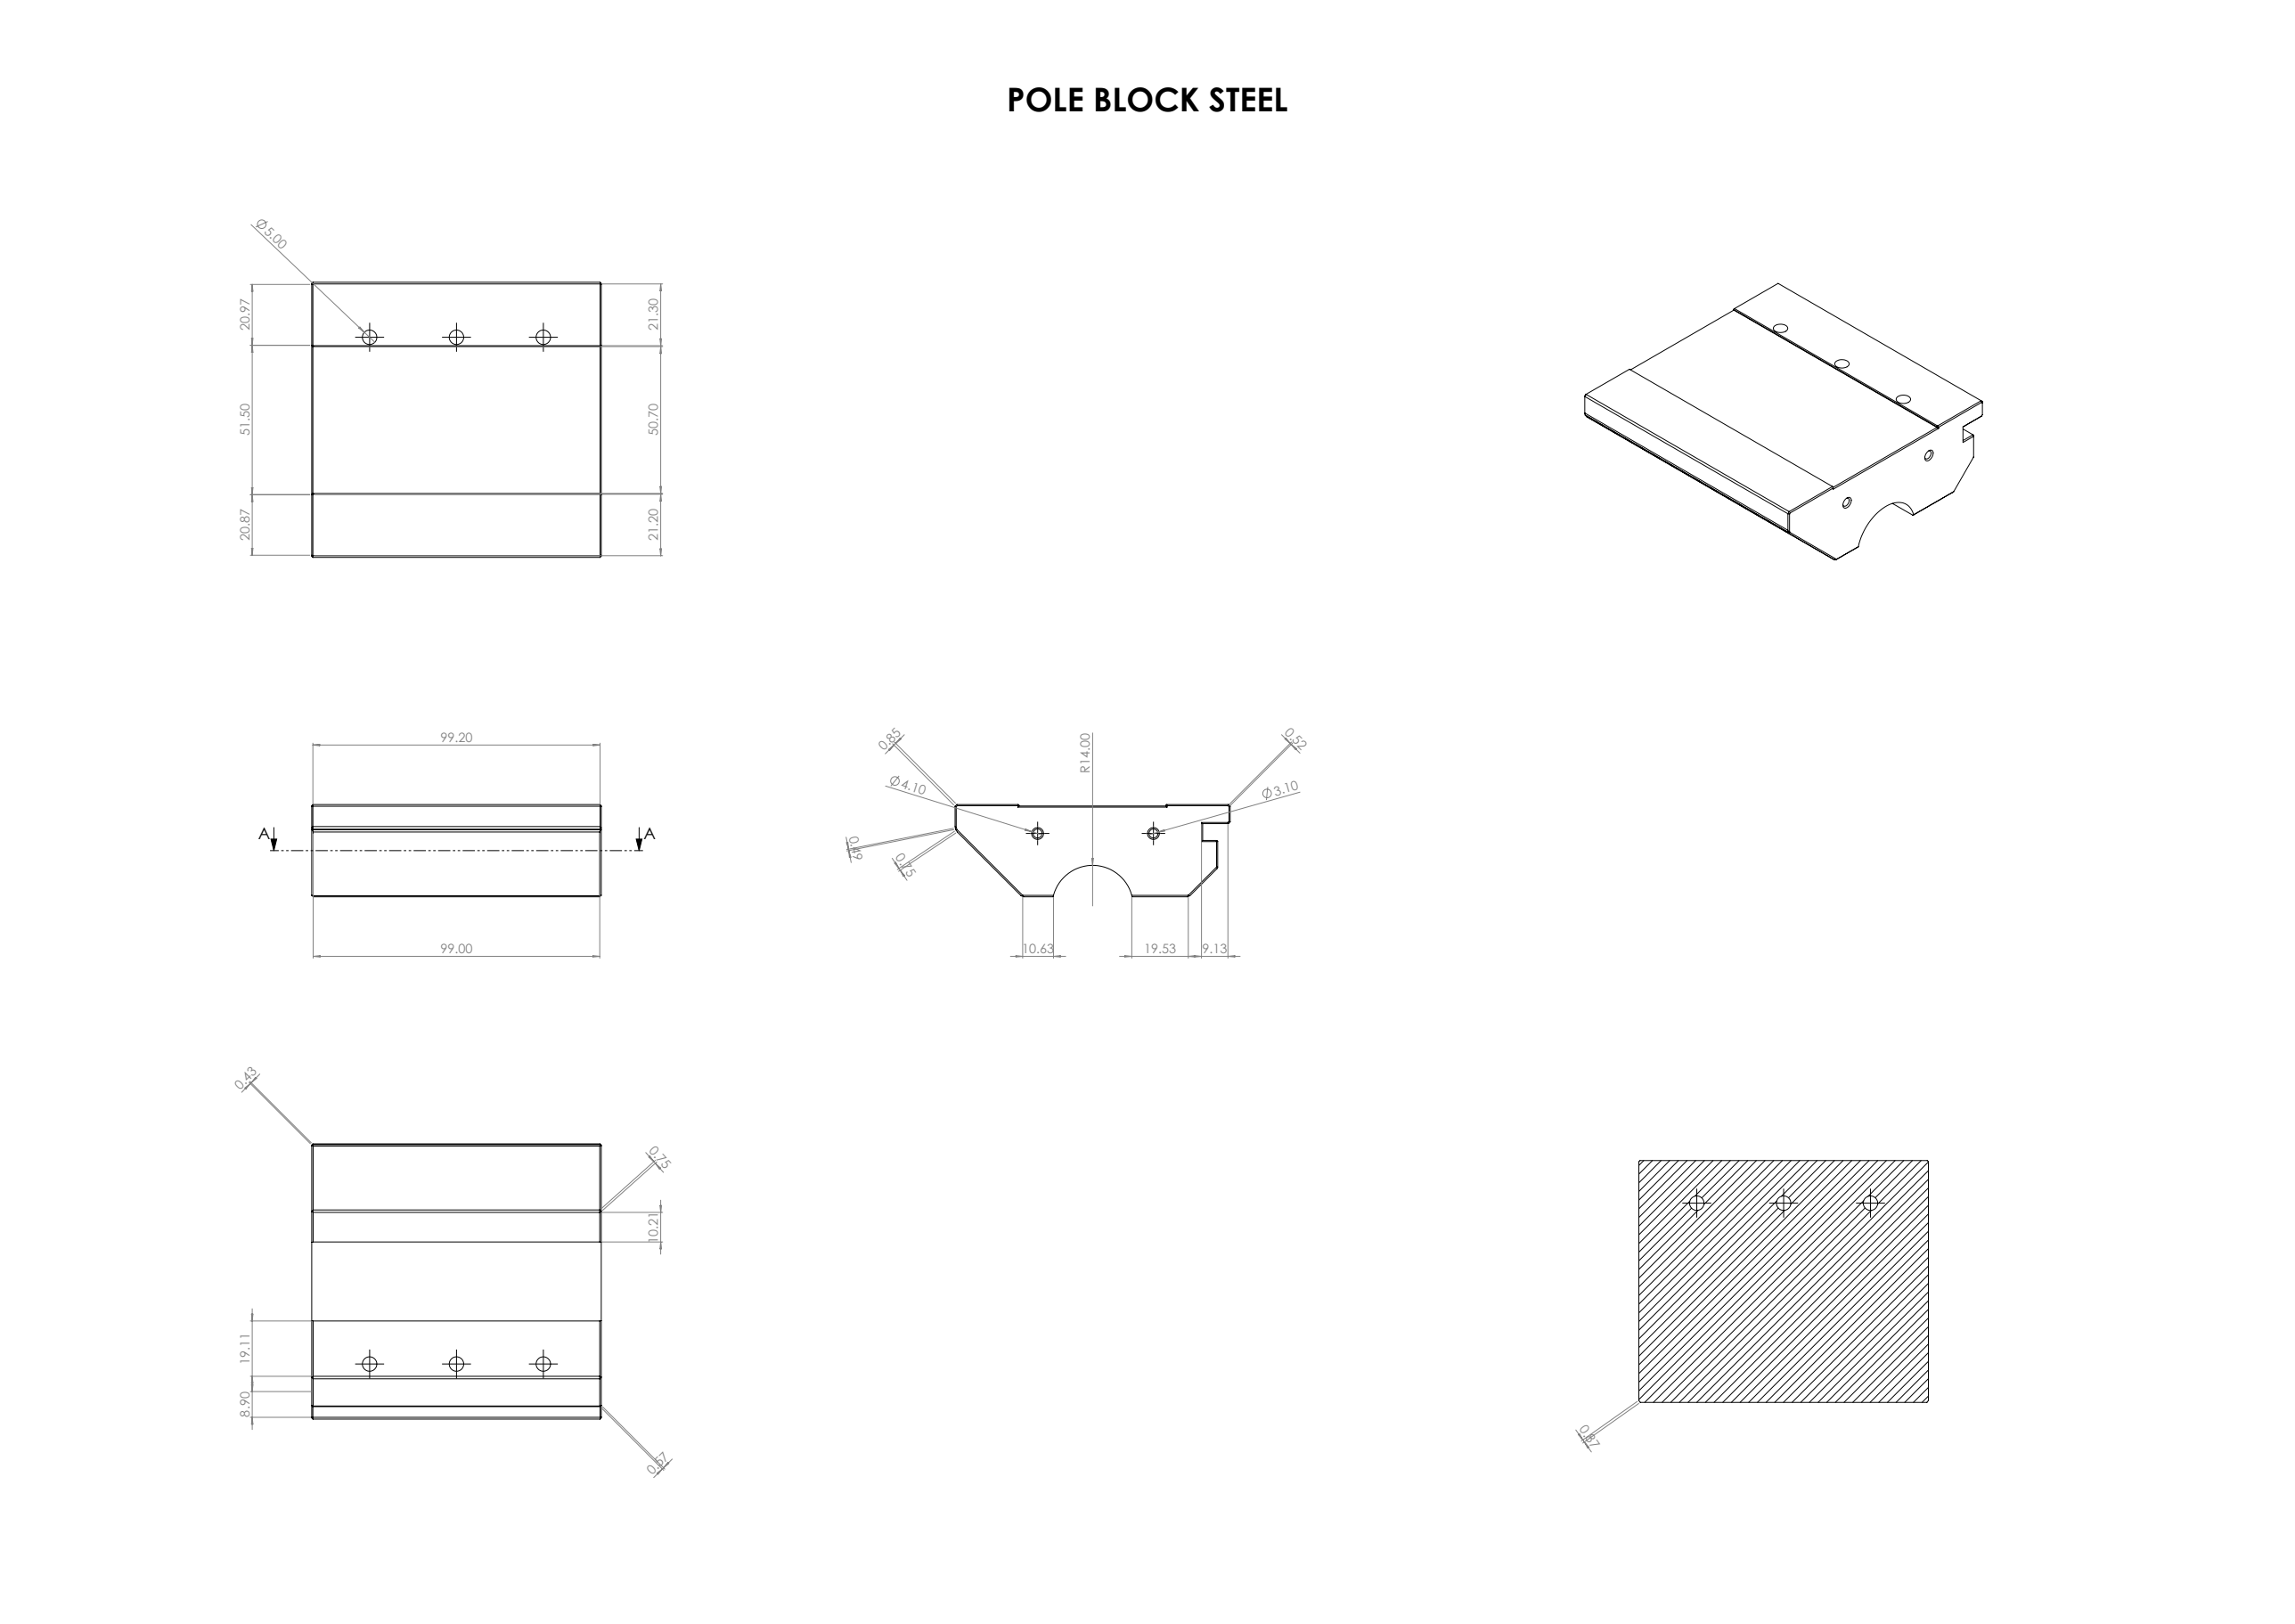
ISO-10303-21;
HEADER;
/* Generated by software containing ST-Developer
 * from STEP Tools, Inc. (www.steptools.com) 
 */

FILE_DESCRIPTION(
/* description */ (''),
/* implementation_level */ '2;1');

FILE_NAME(
/* name */ '01_Pole_Block_Steel.step',
/* time_stamp */ '2026-10-21T01:59:45-07:00',
/* author */ (''),
/* organization */ (''),
/* preprocessor_version */ 'ST-DEVELOPER v20.2',
/* originating_system */ 'Autodesk Translation Framework v15.15.0.0',
/* authorisation */ '');

FILE_SCHEMA (('AUTOMOTIVE_DESIGN { 1 0 10303 214 3 1 1 }'));
ENDSEC;

DATA;
#10=MECHANICAL_DESIGN_GEOMETRIC_PRESENTATION_REPRESENTATION('',(#467,#468,#469,#470,#471,#472),#18281);
#408=CONICAL_SURFACE('',#9545,1.8,0.785398163397447);
#409=CONICAL_SURFACE('',#9553,1.8,0.785398163397447);
#410=CONICAL_SURFACE('',#9564,1.8,0.785398163397439);
#411=CONICAL_SURFACE('',#9572,1.8,0.785398163397439);
#441=SHAPE_REPRESENTATION_RELATIONSHIP('SRR','None',#18343,#454);
#454=ADVANCED_BREP_SHAPE_REPRESENTATION('',(#485),#18272);
#467=STYLED_ITEM('',(#18453),#8809);
#468=STYLED_ITEM('',(#18453),#8821);
#469=STYLED_ITEM('',(#18453),#8888);
#470=STYLED_ITEM('',(#18453),#8889);
#471=STYLED_ITEM('',(#18453),#8890);
#472=STYLED_ITEM('',(#18453),#485);
#485=MANIFOLD_SOLID_BREP('Body1',#9089);
#517=CYLINDRICAL_SURFACE('',#9551,1.55);
#518=CYLINDRICAL_SURFACE('',#9555,1.55);
#519=CYLINDRICAL_SURFACE('',#9570,1.55);
#520=CYLINDRICAL_SURFACE('',#9574,1.55);
#521=CYLINDRICAL_SURFACE('',#9598,14.);
#522=CYLINDRICAL_SURFACE('',#9660,2.5);
#523=CYLINDRICAL_SURFACE('',#9661,2.5);
#524=CYLINDRICAL_SURFACE('',#9662,2.5);
#608=FACE_BOUND('',#1640,.T.);
#609=FACE_BOUND('',#1641,.T.);
#610=FACE_BOUND('',#1654,.T.);
#611=FACE_BOUND('',#1655,.T.);
#612=FACE_BOUND('',#1674,.T.);
#613=FACE_BOUND('',#1675,.T.);
#614=FACE_BOUND('',#1676,.T.);
#615=FACE_BOUND('',#1724,.T.);
#616=FACE_BOUND('',#1725,.T.);
#617=FACE_BOUND('',#1726,.T.);
#713=CIRCLE('',#9546,2.05);
#714=CIRCLE('',#9547,1.55);
#715=CIRCLE('',#9549,14.);
#716=CIRCLE('',#9550,2.05);
#717=CIRCLE('',#9552,1.55);
#718=CIRCLE('',#9554,1.55);
#719=CIRCLE('',#9556,1.55);
#720=CIRCLE('',#9565,2.05);
#721=CIRCLE('',#9566,1.55);
#722=CIRCLE('',#9568,14.);
#723=CIRCLE('',#9569,2.05);
#724=CIRCLE('',#9571,1.55);
#725=CIRCLE('',#9573,1.55);
#726=CIRCLE('',#9575,1.55);
#727=CIRCLE('',#9595,2.5);
#728=CIRCLE('',#9596,2.5);
#729=CIRCLE('',#9597,2.5);
#730=CIRCLE('',#9645,2.5);
#731=CIRCLE('',#9646,2.5);
#732=CIRCLE('',#9647,2.5);
#830=ELLIPSE('',#9579,19.7989898732233,14.);
#831=ELLIPSE('',#9583,19.7989898732235,14.);
#832=ELLIPSE('',#9591,19.7989898732235,14.);
#833=ELLIPSE('',#9593,19.7989898732233,14.);
#1087=FACE_OUTER_BOUND('',#1638,.T.);
#1088=FACE_OUTER_BOUND('',#1639,.T.);
#1089=FACE_OUTER_BOUND('',#1642,.T.);
#1090=FACE_OUTER_BOUND('',#1643,.T.);
#1091=FACE_OUTER_BOUND('',#1644,.T.);
#1092=FACE_OUTER_BOUND('',#1645,.T.);
#1093=FACE_OUTER_BOUND('',#1646,.T.);
#1094=FACE_OUTER_BOUND('',#1647,.T.);
#1095=FACE_OUTER_BOUND('',#1648,.T.);
#1096=FACE_OUTER_BOUND('',#1649,.T.);
#1097=FACE_OUTER_BOUND('',#1650,.T.);
#1098=FACE_OUTER_BOUND('',#1651,.T.);
#1099=FACE_OUTER_BOUND('',#1652,.T.);
#1100=FACE_OUTER_BOUND('',#1653,.T.);
#1101=FACE_OUTER_BOUND('',#1656,.T.);
#1102=FACE_OUTER_BOUND('',#1657,.T.);
#1103=FACE_OUTER_BOUND('',#1658,.T.);
#1104=FACE_OUTER_BOUND('',#1659,.T.);
#1105=FACE_OUTER_BOUND('',#1660,.T.);
#1106=FACE_OUTER_BOUND('',#1661,.T.);
#1107=FACE_OUTER_BOUND('',#1662,.T.);
#1108=FACE_OUTER_BOUND('',#1663,.T.);
#1109=FACE_OUTER_BOUND('',#1664,.T.);
#1110=FACE_OUTER_BOUND('',#1665,.T.);
#1111=FACE_OUTER_BOUND('',#1666,.T.);
#1112=FACE_OUTER_BOUND('',#1667,.T.);
#1113=FACE_OUTER_BOUND('',#1668,.T.);
#1114=FACE_OUTER_BOUND('',#1669,.T.);
#1115=FACE_OUTER_BOUND('',#1670,.T.);
#1116=FACE_OUTER_BOUND('',#1671,.T.);
#1117=FACE_OUTER_BOUND('',#1672,.T.);
#1118=FACE_OUTER_BOUND('',#1673,.T.);
#1119=FACE_OUTER_BOUND('',#1677,.T.);
#1120=FACE_OUTER_BOUND('',#1678,.T.);
#1121=FACE_OUTER_BOUND('',#1679,.T.);
#1122=FACE_OUTER_BOUND('',#1680,.T.);
#1123=FACE_OUTER_BOUND('',#1681,.T.);
#1124=FACE_OUTER_BOUND('',#1682,.T.);
#1125=FACE_OUTER_BOUND('',#1683,.T.);
#1126=FACE_OUTER_BOUND('',#1684,.T.);
#1127=FACE_OUTER_BOUND('',#1685,.T.);
#1128=FACE_OUTER_BOUND('',#1686,.T.);
#1129=FACE_OUTER_BOUND('',#1687,.T.);
#1130=FACE_OUTER_BOUND('',#1688,.T.);
#1131=FACE_OUTER_BOUND('',#1689,.T.);
#1132=FACE_OUTER_BOUND('',#1690,.T.);
#1133=FACE_OUTER_BOUND('',#1691,.T.);
#1134=FACE_OUTER_BOUND('',#1692,.T.);
#1135=FACE_OUTER_BOUND('',#1693,.T.);
#1136=FACE_OUTER_BOUND('',#1694,.T.);
#1137=FACE_OUTER_BOUND('',#1695,.T.);
#1138=FACE_OUTER_BOUND('',#1696,.T.);
#1139=FACE_OUTER_BOUND('',#1697,.T.);
#1140=FACE_OUTER_BOUND('',#1698,.T.);
#1141=FACE_OUTER_BOUND('',#1699,.T.);
#1142=FACE_OUTER_BOUND('',#1700,.T.);
#1143=FACE_OUTER_BOUND('',#1701,.T.);
#1144=FACE_OUTER_BOUND('',#1702,.T.);
#1145=FACE_OUTER_BOUND('',#1703,.T.);
#1146=FACE_OUTER_BOUND('',#1704,.T.);
#1147=FACE_OUTER_BOUND('',#1705,.T.);
#1148=FACE_OUTER_BOUND('',#1706,.T.);
#1149=FACE_OUTER_BOUND('',#1707,.T.);
#1150=FACE_OUTER_BOUND('',#1708,.T.);
#1151=FACE_OUTER_BOUND('',#1709,.T.);
#1152=FACE_OUTER_BOUND('',#1710,.T.);
#1153=FACE_OUTER_BOUND('',#1711,.T.);
#1154=FACE_OUTER_BOUND('',#1712,.T.);
#1155=FACE_OUTER_BOUND('',#1713,.T.);
#1156=FACE_OUTER_BOUND('',#1714,.T.);
#1157=FACE_OUTER_BOUND('',#1715,.T.);
#1158=FACE_OUTER_BOUND('',#1716,.T.);
#1159=FACE_OUTER_BOUND('',#1717,.T.);
#1160=FACE_OUTER_BOUND('',#1718,.T.);
#1161=FACE_OUTER_BOUND('',#1719,.T.);
#1162=FACE_OUTER_BOUND('',#1720,.T.);
#1163=FACE_OUTER_BOUND('',#1721,.T.);
#1164=FACE_OUTER_BOUND('',#1722,.T.);
#1165=FACE_OUTER_BOUND('',#1723,.T.);
#1166=FACE_OUTER_BOUND('',#1727,.T.);
#1167=FACE_OUTER_BOUND('',#1728,.T.);
#1168=FACE_OUTER_BOUND('',#1729,.T.);
#1169=FACE_OUTER_BOUND('',#1730,.T.);
#1170=FACE_OUTER_BOUND('',#1731,.T.);
#1171=FACE_OUTER_BOUND('',#1732,.T.);
#1172=FACE_OUTER_BOUND('',#1733,.T.);
#1173=FACE_OUTER_BOUND('',#1734,.T.);
#1174=FACE_OUTER_BOUND('',#1735,.T.);
#1175=FACE_OUTER_BOUND('',#1736,.T.);
#1176=FACE_OUTER_BOUND('',#1737,.T.);
#1177=FACE_OUTER_BOUND('',#1738,.T.);
#1178=FACE_OUTER_BOUND('',#1739,.T.);
#1179=FACE_OUTER_BOUND('',#1740,.T.);
#1180=FACE_OUTER_BOUND('',#1741,.T.);
#1181=FACE_OUTER_BOUND('',#1742,.T.);
#1638=EDGE_LOOP('',(#6924,#6925,#6926,#6927));
#1639=EDGE_LOOP('',(#6928,#6929,#6930,#6931,#6932,#6933,#6934,#6935,#6936,
#6937,#6938,#6939,#6940,#6941,#6942,#6943,#6944,#6945,#6946,#6947,#6948,
#6949,#6950,#6951));
#1640=EDGE_LOOP('',(#6952));
#1641=EDGE_LOOP('',(#6953));
#1642=EDGE_LOOP('',(#6954,#6955,#6956,#6957));
#1643=EDGE_LOOP('',(#6958,#6959,#6960,#6961));
#1644=EDGE_LOOP('',(#6962,#6963,#6964,#6965));
#1645=EDGE_LOOP('',(#6966,#6967,#6968,#6969,#6970,#6971));
#1646=EDGE_LOOP('',(#6972,#6973,#6974,#6975));
#1647=EDGE_LOOP('',(#6976,#6977,#6978,#6979,#6980,#6981));
#1648=EDGE_LOOP('',(#6982,#6983,#6984,#6985,#6986));
#1649=EDGE_LOOP('',(#6987,#6988,#6989,#6990,#6991,#6992));
#1650=EDGE_LOOP('',(#6993,#6994,#6995,#6996,#6997,#6998));
#1651=EDGE_LOOP('',(#6999,#7000,#7001,#7002,#7003));
#1652=EDGE_LOOP('',(#7004,#7005,#7006,#7007));
#1653=EDGE_LOOP('',(#7008,#7009,#7010,#7011,#7012,#7013,#7014,#7015,#7016,
#7017,#7018,#7019,#7020,#7021,#7022,#7023,#7024,#7025,#7026,#7027,#7028,
#7029,#7030,#7031));
#1654=EDGE_LOOP('',(#7032));
#1655=EDGE_LOOP('',(#7033));
#1656=EDGE_LOOP('',(#7034,#7035,#7036,#7037));
#1657=EDGE_LOOP('',(#7038,#7039,#7040,#7041));
#1658=EDGE_LOOP('',(#7042,#7043,#7044,#7045));
#1659=EDGE_LOOP('',(#7046,#7047,#7048));
#1660=EDGE_LOOP('',(#7049,#7050,#7051,#7052,#7053));
#1661=EDGE_LOOP('',(#7054,#7055,#7056,#7057));
#1662=EDGE_LOOP('',(#7058,#7059,#7060));
#1663=EDGE_LOOP('',(#7061,#7062,#7063,#7064));
#1664=EDGE_LOOP('',(#7065,#7066,#7067,#7068));
#1665=EDGE_LOOP('',(#7069,#7070,#7071,#7072));
#1666=EDGE_LOOP('',(#7073,#7074,#7075));
#1667=EDGE_LOOP('',(#7076,#7077,#7078,#7079,#7080));
#1668=EDGE_LOOP('',(#7081,#7082,#7083));
#1669=EDGE_LOOP('',(#7084,#7085,#7086,#7087));
#1670=EDGE_LOOP('',(#7088,#7089,#7090,#7091,#7092));
#1671=EDGE_LOOP('',(#7093,#7094,#7095,#7096));
#1672=EDGE_LOOP('',(#7097,#7098,#7099,#7100));
#1673=EDGE_LOOP('',(#7101,#7102,#7103,#7104));
#1674=EDGE_LOOP('',(#7105));
#1675=EDGE_LOOP('',(#7106));
#1676=EDGE_LOOP('',(#7107));
#1677=EDGE_LOOP('',(#7108,#7109,#7110,#7111,#7112,#7113,#7114,#7115));
#1678=EDGE_LOOP('',(#7116,#7117,#7118,#7119));
#1679=EDGE_LOOP('',(#7120,#7121,#7122,#7123));
#1680=EDGE_LOOP('',(#7124,#7125,#7126,#7127,#7128));
#1681=EDGE_LOOP('',(#7129,#7130,#7131,#7132));
#1682=EDGE_LOOP('',(#7133,#7134,#7135,#7136));
#1683=EDGE_LOOP('',(#7137,#7138,#7139,#7140));
#1684=EDGE_LOOP('',(#7141,#7142,#7143,#7144));
#1685=EDGE_LOOP('',(#7145,#7146,#7147,#7148));
#1686=EDGE_LOOP('',(#7149,#7150,#7151,#7152));
#1687=EDGE_LOOP('',(#7153,#7154,#7155,#7156));
#1688=EDGE_LOOP('',(#7157,#7158,#7159,#7160));
#1689=EDGE_LOOP('',(#7161,#7162,#7163,#7164));
#1690=EDGE_LOOP('',(#7165,#7166,#7167,#7168));
#1691=EDGE_LOOP('',(#7169,#7170,#7171,#7172));
#1692=EDGE_LOOP('',(#7173,#7174,#7175,#7176));
#1693=EDGE_LOOP('',(#7177,#7178,#7179,#7180));
#1694=EDGE_LOOP('',(#7181,#7182,#7183,#7184));
#1695=EDGE_LOOP('',(#7185,#7186,#7187,#7188));
#1696=EDGE_LOOP('',(#7189,#7190,#7191,#7192));
#1697=EDGE_LOOP('',(#7193,#7194,#7195,#7196));
#1698=EDGE_LOOP('',(#7197,#7198,#7199,#7200));
#1699=EDGE_LOOP('',(#7201,#7202,#7203,#7204));
#1700=EDGE_LOOP('',(#7205,#7206,#7207,#7208));
#1701=EDGE_LOOP('',(#7209,#7210,#7211,#7212));
#1702=EDGE_LOOP('',(#7213,#7214,#7215,#7216,#7217,#7218));
#1703=EDGE_LOOP('',(#7219,#7220,#7221,#7222));
#1704=EDGE_LOOP('',(#7223,#7224,#7225,#7226));
#1705=EDGE_LOOP('',(#7227,#7228,#7229,#7230));
#1706=EDGE_LOOP('',(#7231,#7232,#7233,#7234));
#1707=EDGE_LOOP('',(#7235,#7236,#7237,#7238));
#1708=EDGE_LOOP('',(#7239,#7240,#7241,#7242));
#1709=EDGE_LOOP('',(#7243,#7244,#7245,#7246));
#1710=EDGE_LOOP('',(#7247,#7248,#7249,#7250));
#1711=EDGE_LOOP('',(#7251,#7252,#7253,#7254));
#1712=EDGE_LOOP('',(#7255,#7256,#7257,#7258));
#1713=EDGE_LOOP('',(#7259,#7260,#7261,#7262));
#1714=EDGE_LOOP('',(#7263,#7264,#7265,#7266));
#1715=EDGE_LOOP('',(#7267,#7268,#7269,#7270));
#1716=EDGE_LOOP('',(#7271,#7272,#7273,#7274));
#1717=EDGE_LOOP('',(#7275,#7276,#7277,#7278));
#1718=EDGE_LOOP('',(#7279,#7280,#7281,#7282));
#1719=EDGE_LOOP('',(#7283,#7284,#7285,#7286));
#1720=EDGE_LOOP('',(#7287,#7288,#7289,#7290));
#1721=EDGE_LOOP('',(#7291,#7292,#7293,#7294));
#1722=EDGE_LOOP('',(#7295,#7296,#7297,#7298));
#1723=EDGE_LOOP('',(#7299,#7300,#7301,#7302));
#1724=EDGE_LOOP('',(#7303));
#1725=EDGE_LOOP('',(#7304));
#1726=EDGE_LOOP('',(#7305));
#1727=EDGE_LOOP('',(#7306,#7307,#7308,#7309));
#1728=EDGE_LOOP('',(#7310,#7311,#7312,#7313));
#1729=EDGE_LOOP('',(#7314,#7315,#7316,#7317));
#1730=EDGE_LOOP('',(#7318,#7319,#7320,#7321));
#1731=EDGE_LOOP('',(#7322,#7323,#7324,#7325));
#1732=EDGE_LOOP('',(#7326,#7327,#7328,#7329));
#1733=EDGE_LOOP('',(#7330,#7331,#7332,#7333));
#1734=EDGE_LOOP('',(#7334,#7335,#7336,#7337));
#1735=EDGE_LOOP('',(#7338));
#1736=EDGE_LOOP('',(#7339));
#1737=EDGE_LOOP('',(#7340));
#1738=EDGE_LOOP('',(#7341));
#1739=EDGE_LOOP('',(#7342,#7343,#7344,#7345));
#1740=EDGE_LOOP('',(#7346,#7347,#7348,#7349));
#1741=EDGE_LOOP('',(#7350,#7351,#7352,#7353));
#1742=EDGE_LOOP('',(#7354,#7355,#7356,#7357));
#2357=LINE('',#14001,#3202);
#2358=LINE('',#14006,#3203);
#2359=LINE('',#14008,#3204);
#2360=LINE('',#14010,#3205);
#2361=LINE('',#14012,#3206);
#2362=LINE('',#14014,#3207);
#2363=LINE('',#14016,#3208);
#2364=LINE('',#14018,#3209);
#2365=LINE('',#14020,#3210);
#2366=LINE('',#14022,#3211);
#2367=LINE('',#14024,#3212);
#2368=LINE('',#14026,#3213);
#2369=LINE('',#14028,#3214);
#2370=LINE('',#14030,#3215);
#2371=LINE('',#14032,#3216);
#2372=LINE('',#14034,#3217);
#2373=LINE('',#14036,#3218);
#2374=LINE('',#14038,#3219);
#2375=LINE('',#14040,#3220);
#2376=LINE('',#14042,#3221);
#2377=LINE('',#14044,#3222);
#2378=LINE('',#14046,#3223);
#2379=LINE('',#14048,#3224);
#2380=LINE('',#14051,#3225);
#2381=LINE('',#14056,#3226);
#2382=LINE('',#14060,#3227);
#2383=LINE('',#14064,#3228);
#2384=LINE('',#14069,#3229);
#2385=LINE('',#14071,#3230);
#2386=LINE('',#14073,#3231);
#2387=LINE('',#14075,#3232);
#2388=LINE('',#14077,#3233);
#2389=LINE('',#14078,#3234);
#2390=LINE('',#14081,#3235);
#2391=LINE('',#14083,#3236);
#2392=LINE('',#14084,#3237);
#2393=LINE('',#14087,#3238);
#2394=LINE('',#14089,#3239);
#2395=LINE('',#14091,#3240);
#2396=LINE('',#14092,#3241);
#2397=LINE('',#14095,#3242);
#2398=LINE('',#14097,#3243);
#2399=LINE('',#14098,#3244);
#2400=LINE('',#14101,#3245);
#2401=LINE('',#14103,#3246);
#2402=LINE('',#14105,#3247);
#2403=LINE('',#14106,#3248);
#2404=LINE('',#14108,#3249);
#2405=LINE('',#14109,#3250);
#2406=LINE('',#14112,#3251);
#2407=LINE('',#14113,#3252);
#2408=LINE('',#14118,#3253);
#2409=LINE('',#14122,#3254);
#2410=LINE('',#14126,#3255);
#2411=LINE('',#14128,#3256);
#2412=LINE('',#14130,#3257);
#2413=LINE('',#14132,#3258);
#2414=LINE('',#14134,#3259);
#2415=LINE('',#14136,#3260);
#2416=LINE('',#14138,#3261);
#2417=LINE('',#14140,#3262);
#2418=LINE('',#14142,#3263);
#2419=LINE('',#14144,#3264);
#2420=LINE('',#14146,#3265);
#2421=LINE('',#14148,#3266);
#2422=LINE('',#14150,#3267);
#2423=LINE('',#14152,#3268);
#2424=LINE('',#14154,#3269);
#2425=LINE('',#14156,#3270);
#2426=LINE('',#14158,#3271);
#2427=LINE('',#14160,#3272);
#2428=LINE('',#14162,#3273);
#2429=LINE('',#14163,#3274);
#2430=LINE('',#14168,#3275);
#2431=LINE('',#14172,#3276);
#2432=LINE('',#14176,#3277);
#2433=LINE('',#14181,#3278);
#2434=LINE('',#14182,#3279);
#2435=LINE('',#14183,#3280);
#2436=LINE('',#14185,#3281);
#2437=LINE('',#14189,#3282);
#2438=LINE('',#14192,#3283);
#2439=LINE('',#14193,#3284);
#2440=LINE('',#14195,#3285);
#2441=LINE('',#14196,#3286);
#2442=LINE('',#14200,#3287);
#2443=LINE('',#14204,#3288);
#2444=LINE('',#14206,#3289);
#2445=LINE('',#14207,#3290);
#2446=LINE('',#14211,#3291);
#2447=LINE('',#14212,#3292);
#2448=LINE('',#14213,#3293);
#2449=LINE('',#14216,#3294);
#2450=LINE('',#14218,#3295);
#2451=LINE('',#14219,#3296);
#2452=LINE('',#14221,#3297);
#2453=LINE('',#14222,#3298);
#2454=LINE('',#14225,#3299);
#2455=LINE('',#14227,#3300);
#2456=LINE('',#14228,#3301);
#2457=LINE('',#14232,#3302);
#2458=LINE('',#14236,#3303);
#2459=LINE('',#14238,#3304);
#2460=LINE('',#14246,#3305);
#2461=LINE('',#14249,#3306);
#2462=LINE('',#14250,#3307);
#2463=LINE('',#14254,#3308);
#2464=LINE('',#14255,#3309);
#2465=LINE('',#14256,#3310);
#2466=LINE('',#14259,#3311);
#2467=LINE('',#14260,#3312);
#2468=LINE('',#14263,#3313);
#2469=LINE('',#14264,#3314);
#2470=LINE('',#14267,#3315);
#2471=LINE('',#14268,#3316);
#2472=LINE('',#14271,#3317);
#2473=LINE('',#14272,#3318);
#2474=LINE('',#14275,#3319);
#2475=LINE('',#14276,#3320);
#2476=LINE('',#14278,#3321);
#2477=LINE('',#14281,#3322);
#2478=LINE('',#14282,#3323);
#2479=LINE('',#14285,#3324);
#2480=LINE('',#14286,#3325);
#2481=LINE('',#14289,#3326);
#2482=LINE('',#14290,#3327);
#2483=LINE('',#14293,#3328);
#2484=LINE('',#14294,#3329);
#2485=LINE('',#14297,#3330);
#2486=LINE('',#14298,#3331);
#2487=LINE('',#14301,#3332);
#2488=LINE('',#14302,#3333);
#2489=LINE('',#14305,#3334);
#2490=LINE('',#14306,#3335);
#2491=LINE('',#14309,#3336);
#2492=LINE('',#14310,#3337);
#2493=LINE('',#14313,#3338);
#2494=LINE('',#14314,#3339);
#2495=LINE('',#14316,#3340);
#2496=LINE('',#14319,#3341);
#2497=LINE('',#14321,#3342);
#2498=LINE('',#14322,#3343);
#2499=LINE('',#14325,#3344);
#2500=LINE('',#14326,#3345);
#2501=LINE('',#14329,#3346);
#2502=LINE('',#14330,#3347);
#2503=LINE('',#14333,#3348);
#2504=LINE('',#14334,#3349);
#2505=LINE('',#14337,#3350);
#2506=LINE('',#14338,#3351);
#2507=LINE('',#14341,#3352);
#2508=LINE('',#14342,#3353);
#2509=LINE('',#14344,#3354);
#2510=LINE('',#14345,#3355);
#2511=LINE('',#14348,#3356);
#2512=LINE('',#14350,#3357);
#2513=LINE('',#14352,#3358);
#2514=LINE('',#14354,#3359);
#2515=LINE('',#14356,#3360);
#2516=LINE('',#14358,#3361);
#2517=LINE('',#14360,#3362);
#2518=LINE('',#14363,#3363);
#2519=LINE('',#14364,#3364);
#2520=LINE('',#14367,#3365);
#2521=LINE('',#14368,#3366);
#2522=LINE('',#14371,#3367);
#2523=LINE('',#14372,#3368);
#2524=LINE('',#14375,#3369);
#2525=LINE('',#14376,#3370);
#2526=LINE('',#14379,#3371);
#2527=LINE('',#14380,#3372);
#2528=LINE('',#14383,#3373);
#2529=LINE('',#14385,#3374);
#2530=LINE('',#14386,#3375);
#2531=LINE('',#14389,#3376);
#2532=LINE('',#14390,#3377);
#2533=LINE('',#14393,#3378);
#2534=LINE('',#14394,#3379);
#2535=LINE('',#14396,#3380);
#2536=LINE('',#14398,#3381);
#2537=LINE('',#14400,#3382);
#2538=LINE('',#14402,#3383);
#2539=LINE('',#14404,#3384);
#2540=LINE('',#14412,#3385);
#2541=LINE('',#14414,#3386);
#2542=LINE('',#14416,#3387);
#2543=LINE('',#14418,#3388);
#2544=LINE('',#14420,#3389);
#2545=LINE('',#14422,#3390);
#2546=LINE('',#14424,#3391);
#2547=LINE('',#14431,#3392);
#2548=LINE('',#14433,#3393);
#2549=LINE('',#14435,#3394);
#3202=VECTOR('',#11001,1.8);
#3203=VECTOR('',#11006,10.);
#3204=VECTOR('',#11007,10.);
#3205=VECTOR('',#11008,10.);
#3206=VECTOR('',#11009,10.);
#3207=VECTOR('',#11010,10.);
#3208=VECTOR('',#11011,10.);
#3209=VECTOR('',#11012,10.);
#3210=VECTOR('',#11013,10.);
#3211=VECTOR('',#11014,10.);
#3212=VECTOR('',#11015,10.);
#3213=VECTOR('',#11016,10.);
#3214=VECTOR('',#11017,10.);
#3215=VECTOR('',#11018,10.);
#3216=VECTOR('',#11019,10.);
#3217=VECTOR('',#11020,10.);
#3218=VECTOR('',#11021,10.);
#3219=VECTOR('',#11022,10.);
#3220=VECTOR('',#11023,10.);
#3221=VECTOR('',#11024,10.);
#3222=VECTOR('',#11025,10.);
#3223=VECTOR('',#11026,10.);
#3224=VECTOR('',#11027,10.);
#3225=VECTOR('',#11030,10.);
#3226=VECTOR('',#11035,1.55);
#3227=VECTOR('',#11040,1.8);
#3228=VECTOR('',#11045,1.55);
#3229=VECTOR('',#11050,10.);
#3230=VECTOR('',#11051,10.);
#3231=VECTOR('',#11052,10.);
#3232=VECTOR('',#11053,10.);
#3233=VECTOR('',#11054,10.);
#3234=VECTOR('',#11055,10.);
#3235=VECTOR('',#11058,10.);
#3236=VECTOR('',#11059,10.);
#3237=VECTOR('',#11060,10.);
#3238=VECTOR('',#11063,10.);
#3239=VECTOR('',#11064,10.);
#3240=VECTOR('',#11065,10.);
#3241=VECTOR('',#11066,10.);
#3242=VECTOR('',#11069,10.);
#3243=VECTOR('',#11070,10.);
#3244=VECTOR('',#11071,10.);
#3245=VECTOR('',#11074,10.);
#3246=VECTOR('',#11075,10.);
#3247=VECTOR('',#11076,10.);
#3248=VECTOR('',#11077,10.);
#3249=VECTOR('',#11080,10.);
#3250=VECTOR('',#11081,10.);
#3251=VECTOR('',#11084,10.);
#3252=VECTOR('',#11085,10.);
#3253=VECTOR('',#11090,1.8);
#3254=VECTOR('',#11095,10.);
#3255=VECTOR('',#11098,10.);
#3256=VECTOR('',#11099,10.);
#3257=VECTOR('',#11100,10.);
#3258=VECTOR('',#11101,10.);
#3259=VECTOR('',#11102,10.);
#3260=VECTOR('',#11103,10.);
#3261=VECTOR('',#11104,10.);
#3262=VECTOR('',#11105,10.);
#3263=VECTOR('',#11106,10.);
#3264=VECTOR('',#11107,10.);
#3265=VECTOR('',#11108,10.);
#3266=VECTOR('',#11109,10.);
#3267=VECTOR('',#11110,10.);
#3268=VECTOR('',#11111,10.);
#3269=VECTOR('',#11112,10.);
#3270=VECTOR('',#11113,10.);
#3271=VECTOR('',#11114,10.);
#3272=VECTOR('',#11115,10.);
#3273=VECTOR('',#11116,10.);
#3274=VECTOR('',#11117,10.);
#3275=VECTOR('',#11122,1.55);
#3276=VECTOR('',#11127,1.8);
#3277=VECTOR('',#11132,1.55);
#3278=VECTOR('',#11137,10.);
#3279=VECTOR('',#11138,10.);
#3280=VECTOR('',#11139,10.);
#3281=VECTOR('',#11142,10.);
#3282=VECTOR('',#11147,10.);
#3283=VECTOR('',#11150,10.);
#3284=VECTOR('',#11151,10.);
#3285=VECTOR('',#11154,10.);
#3286=VECTOR('',#11155,10.);
#3287=VECTOR('',#11160,10.);
#3288=VECTOR('',#11165,10.);
#3289=VECTOR('',#11166,10.);
#3290=VECTOR('',#11167,10.);
#3291=VECTOR('',#11170,10.);
#3292=VECTOR('',#11171,10.);
#3293=VECTOR('',#11172,10.);
#3294=VECTOR('',#11175,10.);
#3295=VECTOR('',#11176,10.);
#3296=VECTOR('',#11177,10.);
#3297=VECTOR('',#11180,10.);
#3298=VECTOR('',#11181,10.);
#3299=VECTOR('',#11184,10.);
#3300=VECTOR('',#11185,10.);
#3301=VECTOR('',#11186,10.);
#3302=VECTOR('',#11191,10.);
#3303=VECTOR('',#11196,10.);
#3304=VECTOR('',#11199,10.);
#3305=VECTOR('',#11208,10.);
#3306=VECTOR('',#11211,10.);
#3307=VECTOR('',#11212,10.);
#3308=VECTOR('',#11215,10.);
#3309=VECTOR('',#11216,10.);
#3310=VECTOR('',#11217,10.);
#3311=VECTOR('',#11220,10.);
#3312=VECTOR('',#11221,10.);
#3313=VECTOR('',#11224,10.);
#3314=VECTOR('',#11225,10.);
#3315=VECTOR('',#11228,10.);
#3316=VECTOR('',#11229,10.);
#3317=VECTOR('',#11232,10.);
#3318=VECTOR('',#11233,10.);
#3319=VECTOR('',#11236,10.);
#3320=VECTOR('',#11237,10.);
#3321=VECTOR('',#11240,10.);
#3322=VECTOR('',#11243,10.);
#3323=VECTOR('',#11244,10.);
#3324=VECTOR('',#11247,10.);
#3325=VECTOR('',#11248,10.);
#3326=VECTOR('',#11251,10.);
#3327=VECTOR('',#11252,10.);
#3328=VECTOR('',#11255,10.);
#3329=VECTOR('',#11256,10.);
#3330=VECTOR('',#11259,10.);
#3331=VECTOR('',#11260,10.);
#3332=VECTOR('',#11263,10.);
#3333=VECTOR('',#11264,10.);
#3334=VECTOR('',#11267,10.);
#3335=VECTOR('',#11268,10.);
#3336=VECTOR('',#11271,10.);
#3337=VECTOR('',#11272,10.);
#3338=VECTOR('',#11275,10.);
#3339=VECTOR('',#11276,10.);
#3340=VECTOR('',#11279,10.);
#3341=VECTOR('',#11282,10.);
#3342=VECTOR('',#11283,10.);
#3343=VECTOR('',#11284,10.);
#3344=VECTOR('',#11287,10.);
#3345=VECTOR('',#11288,10.);
#3346=VECTOR('',#11291,10.);
#3347=VECTOR('',#11292,10.);
#3348=VECTOR('',#11295,10.);
#3349=VECTOR('',#11296,10.);
#3350=VECTOR('',#11299,10.);
#3351=VECTOR('',#11300,10.);
#3352=VECTOR('',#11303,10.);
#3353=VECTOR('',#11304,10.);
#3354=VECTOR('',#11307,10.);
#3355=VECTOR('',#11308,10.);
#3356=VECTOR('',#11313,10.);
#3357=VECTOR('',#11316,10.);
#3358=VECTOR('',#11319,10.);
#3359=VECTOR('',#11322,10.);
#3360=VECTOR('',#11325,10.);
#3361=VECTOR('',#11328,10.);
#3362=VECTOR('',#11331,10.);
#3363=VECTOR('',#11334,10.);
#3364=VECTOR('',#11335,10.);
#3365=VECTOR('',#11338,10.);
#3366=VECTOR('',#11339,10.);
#3367=VECTOR('',#11342,10.);
#3368=VECTOR('',#11343,10.);
#3369=VECTOR('',#11346,10.);
#3370=VECTOR('',#11347,10.);
#3371=VECTOR('',#11350,10.);
#3372=VECTOR('',#11351,10.);
#3373=VECTOR('',#11354,10.);
#3374=VECTOR('',#11355,10.);
#3375=VECTOR('',#11356,10.);
#3376=VECTOR('',#11359,10.);
#3377=VECTOR('',#11360,10.);
#3378=VECTOR('',#11363,10.);
#3379=VECTOR('',#11364,10.);
#3380=VECTOR('',#11367,10.);
#3381=VECTOR('',#11370,10.);
#3382=VECTOR('',#11373,10.);
#3383=VECTOR('',#11376,10.);
#3384=VECTOR('',#11379,10.);
#3385=VECTOR('',#11388,10.);
#3386=VECTOR('',#11391,10.);
#3387=VECTOR('',#11394,10.);
#3388=VECTOR('',#11397,10.);
#3389=VECTOR('',#11400,10.);
#3390=VECTOR('',#11403,10.);
#3391=VECTOR('',#11406,10.);
#3392=VECTOR('',#11419,2.5);
#3393=VECTOR('',#11422,2.5);
#3394=VECTOR('',#11425,2.5);
#4008=VERTEX_POINT('',#13998);
#4009=VERTEX_POINT('',#14000);
#4010=VERTEX_POINT('',#14004);
#4011=VERTEX_POINT('',#14005);
#4012=VERTEX_POINT('',#14007);
#4013=VERTEX_POINT('',#14009);
#4014=VERTEX_POINT('',#14011);
#4015=VERTEX_POINT('',#14013);
#4016=VERTEX_POINT('',#14015);
#4017=VERTEX_POINT('',#14017);
#4018=VERTEX_POINT('',#14019);
#4019=VERTEX_POINT('',#14021);
#4020=VERTEX_POINT('',#14023);
#4021=VERTEX_POINT('',#14025);
#4022=VERTEX_POINT('',#14027);
#4023=VERTEX_POINT('',#14029);
#4024=VERTEX_POINT('',#14031);
#4025=VERTEX_POINT('',#14033);
#4026=VERTEX_POINT('',#14035);
#4027=VERTEX_POINT('',#14037);
#4028=VERTEX_POINT('',#14039);
#4029=VERTEX_POINT('',#14041);
#4030=VERTEX_POINT('',#14043);
#4031=VERTEX_POINT('',#14045);
#4032=VERTEX_POINT('',#14047);
#4033=VERTEX_POINT('',#14049);
#4034=VERTEX_POINT('',#14052);
#4035=VERTEX_POINT('',#14055);
#4036=VERTEX_POINT('',#14059);
#4037=VERTEX_POINT('',#14063);
#4038=VERTEX_POINT('',#14067);
#4039=VERTEX_POINT('',#14068);
#4040=VERTEX_POINT('',#14070);
#4041=VERTEX_POINT('',#14072);
#4042=VERTEX_POINT('',#14074);
#4043=VERTEX_POINT('',#14076);
#4044=VERTEX_POINT('',#14080);
#4045=VERTEX_POINT('',#14082);
#4046=VERTEX_POINT('',#14086);
#4047=VERTEX_POINT('',#14088);
#4048=VERTEX_POINT('',#14090);
#4049=VERTEX_POINT('',#14094);
#4050=VERTEX_POINT('',#14096);
#4051=VERTEX_POINT('',#14100);
#4052=VERTEX_POINT('',#14102);
#4053=VERTEX_POINT('',#14104);
#4054=VERTEX_POINT('',#14111);
#4055=VERTEX_POINT('',#14115);
#4056=VERTEX_POINT('',#14117);
#4057=VERTEX_POINT('',#14121);
#4058=VERTEX_POINT('',#14123);
#4059=VERTEX_POINT('',#14125);
#4060=VERTEX_POINT('',#14127);
#4061=VERTEX_POINT('',#14129);
#4062=VERTEX_POINT('',#14131);
#4063=VERTEX_POINT('',#14133);
#4064=VERTEX_POINT('',#14135);
#4065=VERTEX_POINT('',#14137);
#4066=VERTEX_POINT('',#14139);
#4067=VERTEX_POINT('',#14141);
#4068=VERTEX_POINT('',#14143);
#4069=VERTEX_POINT('',#14145);
#4070=VERTEX_POINT('',#14147);
#4071=VERTEX_POINT('',#14149);
#4072=VERTEX_POINT('',#14151);
#4073=VERTEX_POINT('',#14153);
#4074=VERTEX_POINT('',#14155);
#4075=VERTEX_POINT('',#14157);
#4076=VERTEX_POINT('',#14159);
#4077=VERTEX_POINT('',#14161);
#4078=VERTEX_POINT('',#14164);
#4079=VERTEX_POINT('',#14167);
#4080=VERTEX_POINT('',#14171);
#4081=VERTEX_POINT('',#14175);
#4082=VERTEX_POINT('',#14179);
#4083=VERTEX_POINT('',#14180);
#4084=VERTEX_POINT('',#14187);
#4085=VERTEX_POINT('',#14191);
#4086=VERTEX_POINT('',#14198);
#4087=VERTEX_POINT('',#14203);
#4088=VERTEX_POINT('',#14205);
#4089=VERTEX_POINT('',#14209);
#4090=VERTEX_POINT('',#14210);
#4091=VERTEX_POINT('',#14215);
#4092=VERTEX_POINT('',#14217);
#4093=VERTEX_POINT('',#14224);
#4094=VERTEX_POINT('',#14226);
#4095=VERTEX_POINT('',#14230);
#4096=VERTEX_POINT('',#14234);
#4097=VERTEX_POINT('',#14239);
#4098=VERTEX_POINT('',#14241);
#4099=VERTEX_POINT('',#14243);
#4100=VERTEX_POINT('',#14248);
#4101=VERTEX_POINT('',#14252);
#4102=VERTEX_POINT('',#14253);
#4103=VERTEX_POINT('',#14258);
#4104=VERTEX_POINT('',#14262);
#4105=VERTEX_POINT('',#14266);
#4106=VERTEX_POINT('',#14270);
#4107=VERTEX_POINT('',#14274);
#4108=VERTEX_POINT('',#14280);
#4109=VERTEX_POINT('',#14284);
#4110=VERTEX_POINT('',#14288);
#4111=VERTEX_POINT('',#14292);
#4112=VERTEX_POINT('',#14296);
#4113=VERTEX_POINT('',#14300);
#4114=VERTEX_POINT('',#14304);
#4115=VERTEX_POINT('',#14308);
#4116=VERTEX_POINT('',#14312);
#4117=VERTEX_POINT('',#14318);
#4118=VERTEX_POINT('',#14320);
#4119=VERTEX_POINT('',#14324);
#4120=VERTEX_POINT('',#14328);
#4121=VERTEX_POINT('',#14332);
#4122=VERTEX_POINT('',#14336);
#4123=VERTEX_POINT('',#14340);
#4124=VERTEX_POINT('',#14362);
#4125=VERTEX_POINT('',#14366);
#4126=VERTEX_POINT('',#14370);
#4127=VERTEX_POINT('',#14374);
#4128=VERTEX_POINT('',#14378);
#4129=VERTEX_POINT('',#14382);
#4130=VERTEX_POINT('',#14384);
#4131=VERTEX_POINT('',#14388);
#4132=VERTEX_POINT('',#14392);
#4133=VERTEX_POINT('',#14405);
#4134=VERTEX_POINT('',#14407);
#4135=VERTEX_POINT('',#14409);
#5034=EDGE_CURVE('',#4008,#4008,#713,.T.);
#5035=EDGE_CURVE('',#4008,#4009,#2357,.T.);
#5036=EDGE_CURVE('',#4009,#4009,#714,.T.);
#5037=EDGE_CURVE('',#4010,#4011,#2358,.T.);
#5038=EDGE_CURVE('',#4012,#4010,#2359,.T.);
#5039=EDGE_CURVE('',#4013,#4012,#2360,.T.);
#5040=EDGE_CURVE('',#4014,#4013,#2361,.T.);
#5041=EDGE_CURVE('',#4015,#4014,#2362,.T.);
#5042=EDGE_CURVE('',#4016,#4015,#2363,.T.);
#5043=EDGE_CURVE('',#4017,#4016,#2364,.T.);
#5044=EDGE_CURVE('',#4018,#4017,#2365,.T.);
#5045=EDGE_CURVE('',#4019,#4018,#2366,.T.);
#5046=EDGE_CURVE('',#4020,#4019,#2367,.T.);
#5047=EDGE_CURVE('',#4021,#4020,#2368,.T.);
#5048=EDGE_CURVE('',#4022,#4021,#2369,.T.);
#5049=EDGE_CURVE('',#4023,#4022,#2370,.T.);
#5050=EDGE_CURVE('',#4024,#4023,#2371,.T.);
#5051=EDGE_CURVE('',#4025,#4024,#2372,.T.);
#5052=EDGE_CURVE('',#4026,#4025,#2373,.T.);
#5053=EDGE_CURVE('',#4027,#4026,#2374,.T.);
#5054=EDGE_CURVE('',#4028,#4027,#2375,.T.);
#5055=EDGE_CURVE('',#4029,#4028,#2376,.T.);
#5056=EDGE_CURVE('',#4030,#4029,#2377,.T.);
#5057=EDGE_CURVE('',#4031,#4030,#2378,.T.);
#5058=EDGE_CURVE('',#4032,#4031,#2379,.T.);
#5059=EDGE_CURVE('',#4032,#4033,#715,.T.);
#5060=EDGE_CURVE('',#4011,#4033,#2380,.T.);
#5061=EDGE_CURVE('',#4034,#4034,#716,.T.);
#5062=EDGE_CURVE('',#4009,#4035,#2381,.T.);
#5063=EDGE_CURVE('',#4035,#4035,#717,.T.);
#5064=EDGE_CURVE('',#4034,#4036,#2382,.T.);
#5065=EDGE_CURVE('',#4036,#4036,#718,.T.);
#5066=EDGE_CURVE('',#4036,#4037,#2383,.T.);
#5067=EDGE_CURVE('',#4037,#4037,#719,.T.);
#5068=EDGE_CURVE('',#4038,#4039,#2384,.T.);
#5069=EDGE_CURVE('',#4039,#4040,#2385,.T.);
#5070=EDGE_CURVE('',#4040,#4041,#2386,.T.);
#5071=EDGE_CURVE('',#4041,#4042,#2387,.T.);
#5072=EDGE_CURVE('',#4042,#4043,#2388,.T.);
#5073=EDGE_CURVE('',#4043,#4038,#2389,.T.);
#5074=EDGE_CURVE('',#4044,#4039,#2390,.T.);
#5075=EDGE_CURVE('',#4045,#4044,#2391,.T.);
#5076=EDGE_CURVE('',#4040,#4045,#2392,.T.);
#5077=EDGE_CURVE('',#4046,#4038,#2393,.T.);
#5078=EDGE_CURVE('',#4046,#4047,#2394,.T.);
#5079=EDGE_CURVE('',#4047,#4048,#2395,.T.);
#5080=EDGE_CURVE('',#4044,#4048,#2396,.T.);
#5081=EDGE_CURVE('',#4043,#4049,#2397,.T.);
#5082=EDGE_CURVE('',#4049,#4050,#2398,.T.);
#5083=EDGE_CURVE('',#4050,#4046,#2399,.T.);
#5084=EDGE_CURVE('',#4051,#4045,#2400,.T.);
#5085=EDGE_CURVE('',#4048,#4052,#2401,.T.);
#5086=EDGE_CURVE('',#4052,#4053,#2402,.T.);
#5087=EDGE_CURVE('',#4053,#4051,#2403,.T.);
#5088=EDGE_CURVE('',#4012,#4051,#2404,.T.);
#5089=EDGE_CURVE('',#4041,#4010,#2405,.T.);
#5090=EDGE_CURVE('',#4053,#4054,#2406,.T.);
#5091=EDGE_CURVE('',#4013,#4054,#2407,.T.);
#5092=EDGE_CURVE('',#4055,#4055,#720,.T.);
#5093=EDGE_CURVE('',#4055,#4056,#2408,.T.);
#5094=EDGE_CURVE('',#4056,#4056,#721,.T.);
#5095=EDGE_CURVE('',#4057,#4050,#2409,.T.);
#5096=EDGE_CURVE('',#4057,#4058,#722,.T.);
#5097=EDGE_CURVE('',#4059,#4058,#2410,.T.);
#5098=EDGE_CURVE('',#4060,#4059,#2411,.T.);
#5099=EDGE_CURVE('',#4061,#4060,#2412,.T.);
#5100=EDGE_CURVE('',#4062,#4061,#2413,.T.);
#5101=EDGE_CURVE('',#4063,#4062,#2414,.T.);
#5102=EDGE_CURVE('',#4064,#4063,#2415,.T.);
#5103=EDGE_CURVE('',#4065,#4064,#2416,.T.);
#5104=EDGE_CURVE('',#4066,#4065,#2417,.T.);
#5105=EDGE_CURVE('',#4067,#4066,#2418,.T.);
#5106=EDGE_CURVE('',#4068,#4067,#2419,.T.);
#5107=EDGE_CURVE('',#4069,#4068,#2420,.T.);
#5108=EDGE_CURVE('',#4070,#4069,#2421,.T.);
#5109=EDGE_CURVE('',#4071,#4070,#2422,.T.);
#5110=EDGE_CURVE('',#4072,#4071,#2423,.T.);
#5111=EDGE_CURVE('',#4073,#4072,#2424,.T.);
#5112=EDGE_CURVE('',#4074,#4073,#2425,.T.);
#5113=EDGE_CURVE('',#4075,#4074,#2426,.T.);
#5114=EDGE_CURVE('',#4076,#4075,#2427,.T.);
#5115=EDGE_CURVE('',#4077,#4076,#2428,.T.);
#5116=EDGE_CURVE('',#4047,#4077,#2429,.T.);
#5117=EDGE_CURVE('',#4078,#4078,#723,.T.);
#5118=EDGE_CURVE('',#4056,#4079,#2430,.T.);
#5119=EDGE_CURVE('',#4079,#4079,#724,.T.);
#5120=EDGE_CURVE('',#4078,#4080,#2431,.T.);
#5121=EDGE_CURVE('',#4080,#4080,#725,.T.);
#5122=EDGE_CURVE('',#4080,#4081,#2432,.T.);
#5123=EDGE_CURVE('',#4081,#4081,#726,.T.);
#5124=EDGE_CURVE('',#4082,#4083,#2433,.T.);
#5125=EDGE_CURVE('',#4011,#4082,#2434,.T.);
#5126=EDGE_CURVE('',#4083,#4011,#2435,.T.);
#5127=EDGE_CURVE('',#4082,#4042,#2436,.T.);
#5128=EDGE_CURVE('',#4033,#4084,#830,.T.);
#5129=EDGE_CURVE('',#4084,#4083,#2437,.T.);
#5130=EDGE_CURVE('',#4085,#4049,#2438,.T.);
#5131=EDGE_CURVE('',#4050,#4085,#2439,.T.);
#5132=EDGE_CURVE('',#4049,#4082,#2440,.T.);
#5133=EDGE_CURVE('',#4083,#4085,#2441,.T.);
#5134=EDGE_CURVE('',#4086,#4057,#831,.T.);
#5135=EDGE_CURVE('',#4085,#4086,#2442,.T.);
#5136=EDGE_CURVE('',#4031,#4087,#2443,.T.);
#5137=EDGE_CURVE('',#4088,#4031,#2444,.T.);
#5138=EDGE_CURVE('',#4087,#4088,#2445,.T.);
#5139=EDGE_CURVE('',#4089,#4090,#2446,.T.);
#5140=EDGE_CURVE('',#4090,#4088,#2447,.T.);
#5141=EDGE_CURVE('',#4030,#4089,#2448,.T.);
#5142=EDGE_CURVE('',#4091,#4059,#2449,.T.);
#5143=EDGE_CURVE('',#4092,#4091,#2450,.T.);
#5144=EDGE_CURVE('',#4059,#4092,#2451,.T.);
#5145=EDGE_CURVE('',#4091,#4087,#2452,.T.);
#5146=EDGE_CURVE('',#4088,#4092,#2453,.T.);
#5147=EDGE_CURVE('',#4093,#4060,#2454,.T.);
#5148=EDGE_CURVE('',#4092,#4094,#2455,.T.);
#5149=EDGE_CURVE('',#4094,#4093,#2456,.T.);
#5150=EDGE_CURVE('',#4058,#4095,#832,.T.);
#5151=EDGE_CURVE('',#4095,#4091,#2457,.T.);
#5152=EDGE_CURVE('',#4096,#4032,#833,.T.);
#5153=EDGE_CURVE('',#4087,#4096,#2458,.T.);
#5154=EDGE_CURVE('',#4095,#4096,#2459,.T.);
#5155=EDGE_CURVE('',#4097,#4097,#727,.T.);
#5156=EDGE_CURVE('',#4098,#4098,#728,.T.);
#5157=EDGE_CURVE('',#4099,#4099,#729,.T.);
#5158=EDGE_CURVE('',#4084,#4086,#2460,.T.);
#5159=EDGE_CURVE('',#4093,#4100,#2461,.T.);
#5160=EDGE_CURVE('',#4061,#4100,#2462,.T.);
#5161=EDGE_CURVE('',#4101,#4102,#2463,.T.);
#5162=EDGE_CURVE('',#4102,#4072,#2464,.T.);
#5163=EDGE_CURVE('',#4071,#4101,#2465,.T.);
#5164=EDGE_CURVE('',#4077,#4103,#2466,.T.);
#5165=EDGE_CURVE('',#4103,#4052,#2467,.T.);
#5166=EDGE_CURVE('',#4076,#4104,#2468,.T.);
#5167=EDGE_CURVE('',#4104,#4103,#2469,.T.);
#5168=EDGE_CURVE('',#4075,#4105,#2470,.T.);
#5169=EDGE_CURVE('',#4105,#4104,#2471,.T.);
#5170=EDGE_CURVE('',#4106,#4105,#2472,.T.);
#5171=EDGE_CURVE('',#4074,#4106,#2473,.T.);
#5172=EDGE_CURVE('',#4107,#4106,#2474,.T.);
#5173=EDGE_CURVE('',#4073,#4107,#2475,.T.);
#5174=EDGE_CURVE('',#4102,#4107,#2476,.T.);
#5175=EDGE_CURVE('',#4108,#4101,#2477,.T.);
#5176=EDGE_CURVE('',#4070,#4108,#2478,.T.);
#5177=EDGE_CURVE('',#4109,#4108,#2479,.T.);
#5178=EDGE_CURVE('',#4069,#4109,#2480,.T.);
#5179=EDGE_CURVE('',#4110,#4109,#2481,.T.);
#5180=EDGE_CURVE('',#4068,#4110,#2482,.T.);
#5181=EDGE_CURVE('',#4111,#4110,#2483,.T.);
#5182=EDGE_CURVE('',#4067,#4111,#2484,.T.);
#5183=EDGE_CURVE('',#4112,#4111,#2485,.T.);
#5184=EDGE_CURVE('',#4066,#4112,#2486,.T.);
#5185=EDGE_CURVE('',#4113,#4112,#2487,.T.);
#5186=EDGE_CURVE('',#4065,#4113,#2488,.T.);
#5187=EDGE_CURVE('',#4114,#4113,#2489,.T.);
#5188=EDGE_CURVE('',#4064,#4114,#2490,.T.);
#5189=EDGE_CURVE('',#4115,#4114,#2491,.T.);
#5190=EDGE_CURVE('',#4063,#4115,#2492,.T.);
#5191=EDGE_CURVE('',#4116,#4115,#2493,.T.);
#5192=EDGE_CURVE('',#4062,#4116,#2494,.T.);
#5193=EDGE_CURVE('',#4100,#4116,#2495,.T.);
#5194=EDGE_CURVE('',#4112,#4117,#2496,.T.);
#5195=EDGE_CURVE('',#4118,#4117,#2497,.T.);
#5196=EDGE_CURVE('',#4118,#4111,#2498,.T.);
#5197=EDGE_CURVE('',#4119,#4113,#2499,.T.);
#5198=EDGE_CURVE('',#4117,#4119,#2500,.T.);
#5199=EDGE_CURVE('',#4120,#4114,#2501,.T.);
#5200=EDGE_CURVE('',#4119,#4120,#2502,.T.);
#5201=EDGE_CURVE('',#4121,#4115,#2503,.T.);
#5202=EDGE_CURVE('',#4120,#4121,#2504,.T.);
#5203=EDGE_CURVE('',#4116,#4122,#2505,.T.);
#5204=EDGE_CURVE('',#4121,#4122,#2506,.T.);
#5205=EDGE_CURVE('',#4123,#4100,#2507,.T.);
#5206=EDGE_CURVE('',#4122,#4123,#2508,.T.);
#5207=EDGE_CURVE('',#4123,#4089,#2509,.T.);
#5208=EDGE_CURVE('',#4094,#4090,#2510,.T.);
#5209=EDGE_CURVE('',#4029,#4123,#2511,.T.);
#5210=EDGE_CURVE('',#4028,#4122,#2512,.T.);
#5211=EDGE_CURVE('',#4027,#4121,#2513,.T.);
#5212=EDGE_CURVE('',#4026,#4120,#2514,.T.);
#5213=EDGE_CURVE('',#4025,#4119,#2515,.T.);
#5214=EDGE_CURVE('',#4024,#4117,#2516,.T.);
#5215=EDGE_CURVE('',#4023,#4118,#2517,.T.);
#5216=EDGE_CURVE('',#4022,#4124,#2518,.T.);
#5217=EDGE_CURVE('',#4124,#4118,#2519,.T.);
#5218=EDGE_CURVE('',#4021,#4125,#2520,.T.);
#5219=EDGE_CURVE('',#4125,#4124,#2521,.T.);
#5220=EDGE_CURVE('',#4020,#4126,#2522,.T.);
#5221=EDGE_CURVE('',#4126,#4125,#2523,.T.);
#5222=EDGE_CURVE('',#4019,#4127,#2524,.T.);
#5223=EDGE_CURVE('',#4127,#4126,#2525,.T.);
#5224=EDGE_CURVE('',#4018,#4128,#2526,.T.);
#5225=EDGE_CURVE('',#4128,#4127,#2527,.T.);
#5226=EDGE_CURVE('',#4016,#4129,#2528,.T.);
#5227=EDGE_CURVE('',#4129,#4130,#2529,.T.);
#5228=EDGE_CURVE('',#4130,#4017,#2530,.T.);
#5229=EDGE_CURVE('',#4131,#4129,#2531,.T.);
#5230=EDGE_CURVE('',#4015,#4131,#2532,.T.);
#5231=EDGE_CURVE('',#4132,#4131,#2533,.T.);
#5232=EDGE_CURVE('',#4014,#4132,#2534,.T.);
#5233=EDGE_CURVE('',#4130,#4128,#2535,.T.);
#5234=EDGE_CURVE('',#4054,#4132,#2536,.T.);
#5235=EDGE_CURVE('',#4110,#4124,#2537,.T.);
#5236=EDGE_CURVE('',#4125,#4109,#2538,.T.);
#5237=EDGE_CURVE('',#4108,#4126,#2539,.T.);
#5238=EDGE_CURVE('',#4133,#4133,#730,.T.);
#5239=EDGE_CURVE('',#4134,#4134,#731,.T.);
#5240=EDGE_CURVE('',#4135,#4135,#732,.T.);
#5241=EDGE_CURVE('',#4127,#4101,#2540,.T.);
#5242=EDGE_CURVE('',#4128,#4102,#2541,.T.);
#5243=EDGE_CURVE('',#4130,#4107,#2542,.T.);
#5244=EDGE_CURVE('',#4106,#4129,#2543,.T.);
#5245=EDGE_CURVE('',#4131,#4105,#2544,.T.);
#5246=EDGE_CURVE('',#4104,#4132,#2545,.T.);
#5247=EDGE_CURVE('',#4054,#4103,#2546,.T.);
#5248=EDGE_CURVE('',#4133,#4099,#2547,.T.);
#5249=EDGE_CURVE('',#4134,#4098,#2548,.T.);
#5250=EDGE_CURVE('',#4135,#4097,#2549,.T.);
#6924=ORIENTED_EDGE('',*,*,#5034,.T.);
#6925=ORIENTED_EDGE('',*,*,#5035,.T.);
#6926=ORIENTED_EDGE('',*,*,#5036,.T.);
#6927=ORIENTED_EDGE('',*,*,#5035,.F.);
#6928=ORIENTED_EDGE('',*,*,#5037,.F.);
#6929=ORIENTED_EDGE('',*,*,#5038,.F.);
#6930=ORIENTED_EDGE('',*,*,#5039,.F.);
#6931=ORIENTED_EDGE('',*,*,#5040,.F.);
#6932=ORIENTED_EDGE('',*,*,#5041,.F.);
#6933=ORIENTED_EDGE('',*,*,#5042,.F.);
#6934=ORIENTED_EDGE('',*,*,#5043,.F.);
#6935=ORIENTED_EDGE('',*,*,#5044,.F.);
#6936=ORIENTED_EDGE('',*,*,#5045,.F.);
#6937=ORIENTED_EDGE('',*,*,#5046,.F.);
#6938=ORIENTED_EDGE('',*,*,#5047,.F.);
#6939=ORIENTED_EDGE('',*,*,#5048,.F.);
#6940=ORIENTED_EDGE('',*,*,#5049,.F.);
#6941=ORIENTED_EDGE('',*,*,#5050,.F.);
#6942=ORIENTED_EDGE('',*,*,#5051,.F.);
#6943=ORIENTED_EDGE('',*,*,#5052,.F.);
#6944=ORIENTED_EDGE('',*,*,#5053,.F.);
#6945=ORIENTED_EDGE('',*,*,#5054,.F.);
#6946=ORIENTED_EDGE('',*,*,#5055,.F.);
#6947=ORIENTED_EDGE('',*,*,#5056,.F.);
#6948=ORIENTED_EDGE('',*,*,#5057,.F.);
#6949=ORIENTED_EDGE('',*,*,#5058,.F.);
#6950=ORIENTED_EDGE('',*,*,#5059,.T.);
#6951=ORIENTED_EDGE('',*,*,#5060,.F.);
#6952=ORIENTED_EDGE('',*,*,#5061,.F.);
#6953=ORIENTED_EDGE('',*,*,#5034,.F.);
#6954=ORIENTED_EDGE('',*,*,#5036,.F.);
#6955=ORIENTED_EDGE('',*,*,#5062,.T.);
#6956=ORIENTED_EDGE('',*,*,#5063,.T.);
#6957=ORIENTED_EDGE('',*,*,#5062,.F.);
#6958=ORIENTED_EDGE('',*,*,#5061,.T.);
#6959=ORIENTED_EDGE('',*,*,#5064,.T.);
#6960=ORIENTED_EDGE('',*,*,#5065,.T.);
#6961=ORIENTED_EDGE('',*,*,#5064,.F.);
#6962=ORIENTED_EDGE('',*,*,#5065,.F.);
#6963=ORIENTED_EDGE('',*,*,#5066,.T.);
#6964=ORIENTED_EDGE('',*,*,#5067,.T.);
#6965=ORIENTED_EDGE('',*,*,#5066,.F.);
#6966=ORIENTED_EDGE('',*,*,#5068,.T.);
#6967=ORIENTED_EDGE('',*,*,#5069,.T.);
#6968=ORIENTED_EDGE('',*,*,#5070,.T.);
#6969=ORIENTED_EDGE('',*,*,#5071,.T.);
#6970=ORIENTED_EDGE('',*,*,#5072,.T.);
#6971=ORIENTED_EDGE('',*,*,#5073,.T.);
#6972=ORIENTED_EDGE('',*,*,#5069,.F.);
#6973=ORIENTED_EDGE('',*,*,#5074,.F.);
#6974=ORIENTED_EDGE('',*,*,#5075,.F.);
#6975=ORIENTED_EDGE('',*,*,#5076,.F.);
#6976=ORIENTED_EDGE('',*,*,#5068,.F.);
#6977=ORIENTED_EDGE('',*,*,#5077,.F.);
#6978=ORIENTED_EDGE('',*,*,#5078,.T.);
#6979=ORIENTED_EDGE('',*,*,#5079,.T.);
#6980=ORIENTED_EDGE('',*,*,#5080,.F.);
#6981=ORIENTED_EDGE('',*,*,#5074,.T.);
#6982=ORIENTED_EDGE('',*,*,#5073,.F.);
#6983=ORIENTED_EDGE('',*,*,#5081,.T.);
#6984=ORIENTED_EDGE('',*,*,#5082,.T.);
#6985=ORIENTED_EDGE('',*,*,#5083,.T.);
#6986=ORIENTED_EDGE('',*,*,#5077,.T.);
#6987=ORIENTED_EDGE('',*,*,#5084,.T.);
#6988=ORIENTED_EDGE('',*,*,#5075,.T.);
#6989=ORIENTED_EDGE('',*,*,#5080,.T.);
#6990=ORIENTED_EDGE('',*,*,#5085,.T.);
#6991=ORIENTED_EDGE('',*,*,#5086,.T.);
#6992=ORIENTED_EDGE('',*,*,#5087,.T.);
#6993=ORIENTED_EDGE('',*,*,#5070,.F.);
#6994=ORIENTED_EDGE('',*,*,#5076,.T.);
#6995=ORIENTED_EDGE('',*,*,#5084,.F.);
#6996=ORIENTED_EDGE('',*,*,#5088,.F.);
#6997=ORIENTED_EDGE('',*,*,#5038,.T.);
#6998=ORIENTED_EDGE('',*,*,#5089,.F.);
#6999=ORIENTED_EDGE('',*,*,#5087,.F.);
#7000=ORIENTED_EDGE('',*,*,#5090,.T.);
#7001=ORIENTED_EDGE('',*,*,#5091,.F.);
#7002=ORIENTED_EDGE('',*,*,#5039,.T.);
#7003=ORIENTED_EDGE('',*,*,#5088,.T.);
#7004=ORIENTED_EDGE('',*,*,#5092,.T.);
#7005=ORIENTED_EDGE('',*,*,#5093,.T.);
#7006=ORIENTED_EDGE('',*,*,#5094,.T.);
#7007=ORIENTED_EDGE('',*,*,#5093,.F.);
#7008=ORIENTED_EDGE('',*,*,#5083,.F.);
#7009=ORIENTED_EDGE('',*,*,#5095,.F.);
#7010=ORIENTED_EDGE('',*,*,#5096,.T.);
#7011=ORIENTED_EDGE('',*,*,#5097,.F.);
#7012=ORIENTED_EDGE('',*,*,#5098,.F.);
#7013=ORIENTED_EDGE('',*,*,#5099,.F.);
#7014=ORIENTED_EDGE('',*,*,#5100,.F.);
#7015=ORIENTED_EDGE('',*,*,#5101,.F.);
#7016=ORIENTED_EDGE('',*,*,#5102,.F.);
#7017=ORIENTED_EDGE('',*,*,#5103,.F.);
#7018=ORIENTED_EDGE('',*,*,#5104,.F.);
#7019=ORIENTED_EDGE('',*,*,#5105,.F.);
#7020=ORIENTED_EDGE('',*,*,#5106,.F.);
#7021=ORIENTED_EDGE('',*,*,#5107,.F.);
#7022=ORIENTED_EDGE('',*,*,#5108,.F.);
#7023=ORIENTED_EDGE('',*,*,#5109,.F.);
#7024=ORIENTED_EDGE('',*,*,#5110,.F.);
#7025=ORIENTED_EDGE('',*,*,#5111,.F.);
#7026=ORIENTED_EDGE('',*,*,#5112,.F.);
#7027=ORIENTED_EDGE('',*,*,#5113,.F.);
#7028=ORIENTED_EDGE('',*,*,#5114,.F.);
#7029=ORIENTED_EDGE('',*,*,#5115,.F.);
#7030=ORIENTED_EDGE('',*,*,#5116,.F.);
#7031=ORIENTED_EDGE('',*,*,#5078,.F.);
#7032=ORIENTED_EDGE('',*,*,#5117,.F.);
#7033=ORIENTED_EDGE('',*,*,#5092,.F.);
#7034=ORIENTED_EDGE('',*,*,#5094,.F.);
#7035=ORIENTED_EDGE('',*,*,#5118,.T.);
#7036=ORIENTED_EDGE('',*,*,#5119,.T.);
#7037=ORIENTED_EDGE('',*,*,#5118,.F.);
#7038=ORIENTED_EDGE('',*,*,#5117,.T.);
#7039=ORIENTED_EDGE('',*,*,#5120,.T.);
#7040=ORIENTED_EDGE('',*,*,#5121,.T.);
#7041=ORIENTED_EDGE('',*,*,#5120,.F.);
#7042=ORIENTED_EDGE('',*,*,#5121,.F.);
#7043=ORIENTED_EDGE('',*,*,#5122,.T.);
#7044=ORIENTED_EDGE('',*,*,#5123,.T.);
#7045=ORIENTED_EDGE('',*,*,#5122,.F.);
#7046=ORIENTED_EDGE('',*,*,#5124,.F.);
#7047=ORIENTED_EDGE('',*,*,#5125,.F.);
#7048=ORIENTED_EDGE('',*,*,#5126,.F.);
#7049=ORIENTED_EDGE('',*,*,#5071,.F.);
#7050=ORIENTED_EDGE('',*,*,#5089,.T.);
#7051=ORIENTED_EDGE('',*,*,#5037,.T.);
#7052=ORIENTED_EDGE('',*,*,#5125,.T.);
#7053=ORIENTED_EDGE('',*,*,#5127,.T.);
#7054=ORIENTED_EDGE('',*,*,#5128,.T.);
#7055=ORIENTED_EDGE('',*,*,#5129,.T.);
#7056=ORIENTED_EDGE('',*,*,#5126,.T.);
#7057=ORIENTED_EDGE('',*,*,#5060,.T.);
#7058=ORIENTED_EDGE('',*,*,#5082,.F.);
#7059=ORIENTED_EDGE('',*,*,#5130,.F.);
#7060=ORIENTED_EDGE('',*,*,#5131,.F.);
#7061=ORIENTED_EDGE('',*,*,#5130,.T.);
#7062=ORIENTED_EDGE('',*,*,#5132,.T.);
#7063=ORIENTED_EDGE('',*,*,#5124,.T.);
#7064=ORIENTED_EDGE('',*,*,#5133,.T.);
#7065=ORIENTED_EDGE('',*,*,#5134,.T.);
#7066=ORIENTED_EDGE('',*,*,#5095,.T.);
#7067=ORIENTED_EDGE('',*,*,#5131,.T.);
#7068=ORIENTED_EDGE('',*,*,#5135,.T.);
#7069=ORIENTED_EDGE('',*,*,#5072,.F.);
#7070=ORIENTED_EDGE('',*,*,#5127,.F.);
#7071=ORIENTED_EDGE('',*,*,#5132,.F.);
#7072=ORIENTED_EDGE('',*,*,#5081,.F.);
#7073=ORIENTED_EDGE('',*,*,#5136,.F.);
#7074=ORIENTED_EDGE('',*,*,#5137,.F.);
#7075=ORIENTED_EDGE('',*,*,#5138,.F.);
#7076=ORIENTED_EDGE('',*,*,#5139,.T.);
#7077=ORIENTED_EDGE('',*,*,#5140,.T.);
#7078=ORIENTED_EDGE('',*,*,#5137,.T.);
#7079=ORIENTED_EDGE('',*,*,#5057,.T.);
#7080=ORIENTED_EDGE('',*,*,#5141,.T.);
#7081=ORIENTED_EDGE('',*,*,#5142,.F.);
#7082=ORIENTED_EDGE('',*,*,#5143,.F.);
#7083=ORIENTED_EDGE('',*,*,#5144,.F.);
#7084=ORIENTED_EDGE('',*,*,#5143,.T.);
#7085=ORIENTED_EDGE('',*,*,#5145,.T.);
#7086=ORIENTED_EDGE('',*,*,#5138,.T.);
#7087=ORIENTED_EDGE('',*,*,#5146,.T.);
#7088=ORIENTED_EDGE('',*,*,#5147,.T.);
#7089=ORIENTED_EDGE('',*,*,#5098,.T.);
#7090=ORIENTED_EDGE('',*,*,#5144,.T.);
#7091=ORIENTED_EDGE('',*,*,#5148,.T.);
#7092=ORIENTED_EDGE('',*,*,#5149,.T.);
#7093=ORIENTED_EDGE('',*,*,#5150,.T.);
#7094=ORIENTED_EDGE('',*,*,#5151,.T.);
#7095=ORIENTED_EDGE('',*,*,#5142,.T.);
#7096=ORIENTED_EDGE('',*,*,#5097,.T.);
#7097=ORIENTED_EDGE('',*,*,#5152,.T.);
#7098=ORIENTED_EDGE('',*,*,#5058,.T.);
#7099=ORIENTED_EDGE('',*,*,#5136,.T.);
#7100=ORIENTED_EDGE('',*,*,#5153,.T.);
#7101=ORIENTED_EDGE('',*,*,#5153,.F.);
#7102=ORIENTED_EDGE('',*,*,#5145,.F.);
#7103=ORIENTED_EDGE('',*,*,#5151,.F.);
#7104=ORIENTED_EDGE('',*,*,#5154,.T.);
#7105=ORIENTED_EDGE('',*,*,#5155,.T.);
#7106=ORIENTED_EDGE('',*,*,#5156,.T.);
#7107=ORIENTED_EDGE('',*,*,#5157,.T.);
#7108=ORIENTED_EDGE('',*,*,#5128,.F.);
#7109=ORIENTED_EDGE('',*,*,#5059,.F.);
#7110=ORIENTED_EDGE('',*,*,#5152,.F.);
#7111=ORIENTED_EDGE('',*,*,#5154,.F.);
#7112=ORIENTED_EDGE('',*,*,#5150,.F.);
#7113=ORIENTED_EDGE('',*,*,#5096,.F.);
#7114=ORIENTED_EDGE('',*,*,#5134,.F.);
#7115=ORIENTED_EDGE('',*,*,#5158,.F.);
#7116=ORIENTED_EDGE('',*,*,#5147,.F.);
#7117=ORIENTED_EDGE('',*,*,#5159,.T.);
#7118=ORIENTED_EDGE('',*,*,#5160,.F.);
#7119=ORIENTED_EDGE('',*,*,#5099,.T.);
#7120=ORIENTED_EDGE('',*,*,#5161,.T.);
#7121=ORIENTED_EDGE('',*,*,#5162,.T.);
#7122=ORIENTED_EDGE('',*,*,#5110,.T.);
#7123=ORIENTED_EDGE('',*,*,#5163,.T.);
#7124=ORIENTED_EDGE('',*,*,#5085,.F.);
#7125=ORIENTED_EDGE('',*,*,#5079,.F.);
#7126=ORIENTED_EDGE('',*,*,#5116,.T.);
#7127=ORIENTED_EDGE('',*,*,#5164,.T.);
#7128=ORIENTED_EDGE('',*,*,#5165,.T.);
#7129=ORIENTED_EDGE('',*,*,#5115,.T.);
#7130=ORIENTED_EDGE('',*,*,#5166,.T.);
#7131=ORIENTED_EDGE('',*,*,#5167,.T.);
#7132=ORIENTED_EDGE('',*,*,#5164,.F.);
#7133=ORIENTED_EDGE('',*,*,#5114,.T.);
#7134=ORIENTED_EDGE('',*,*,#5168,.T.);
#7135=ORIENTED_EDGE('',*,*,#5169,.T.);
#7136=ORIENTED_EDGE('',*,*,#5166,.F.);
#7137=ORIENTED_EDGE('',*,*,#5170,.T.);
#7138=ORIENTED_EDGE('',*,*,#5168,.F.);
#7139=ORIENTED_EDGE('',*,*,#5113,.T.);
#7140=ORIENTED_EDGE('',*,*,#5171,.T.);
#7141=ORIENTED_EDGE('',*,*,#5172,.T.);
#7142=ORIENTED_EDGE('',*,*,#5171,.F.);
#7143=ORIENTED_EDGE('',*,*,#5112,.T.);
#7144=ORIENTED_EDGE('',*,*,#5173,.T.);
#7145=ORIENTED_EDGE('',*,*,#5174,.T.);
#7146=ORIENTED_EDGE('',*,*,#5173,.F.);
#7147=ORIENTED_EDGE('',*,*,#5111,.T.);
#7148=ORIENTED_EDGE('',*,*,#5162,.F.);
#7149=ORIENTED_EDGE('',*,*,#5175,.T.);
#7150=ORIENTED_EDGE('',*,*,#5163,.F.);
#7151=ORIENTED_EDGE('',*,*,#5109,.T.);
#7152=ORIENTED_EDGE('',*,*,#5176,.T.);
#7153=ORIENTED_EDGE('',*,*,#5177,.T.);
#7154=ORIENTED_EDGE('',*,*,#5176,.F.);
#7155=ORIENTED_EDGE('',*,*,#5108,.T.);
#7156=ORIENTED_EDGE('',*,*,#5178,.T.);
#7157=ORIENTED_EDGE('',*,*,#5179,.T.);
#7158=ORIENTED_EDGE('',*,*,#5178,.F.);
#7159=ORIENTED_EDGE('',*,*,#5107,.T.);
#7160=ORIENTED_EDGE('',*,*,#5180,.T.);
#7161=ORIENTED_EDGE('',*,*,#5181,.T.);
#7162=ORIENTED_EDGE('',*,*,#5180,.F.);
#7163=ORIENTED_EDGE('',*,*,#5106,.T.);
#7164=ORIENTED_EDGE('',*,*,#5182,.T.);
#7165=ORIENTED_EDGE('',*,*,#5183,.T.);
#7166=ORIENTED_EDGE('',*,*,#5182,.F.);
#7167=ORIENTED_EDGE('',*,*,#5105,.T.);
#7168=ORIENTED_EDGE('',*,*,#5184,.T.);
#7169=ORIENTED_EDGE('',*,*,#5185,.T.);
#7170=ORIENTED_EDGE('',*,*,#5184,.F.);
#7171=ORIENTED_EDGE('',*,*,#5104,.T.);
#7172=ORIENTED_EDGE('',*,*,#5186,.T.);
#7173=ORIENTED_EDGE('',*,*,#5187,.T.);
#7174=ORIENTED_EDGE('',*,*,#5186,.F.);
#7175=ORIENTED_EDGE('',*,*,#5103,.T.);
#7176=ORIENTED_EDGE('',*,*,#5188,.T.);
#7177=ORIENTED_EDGE('',*,*,#5189,.T.);
#7178=ORIENTED_EDGE('',*,*,#5188,.F.);
#7179=ORIENTED_EDGE('',*,*,#5102,.T.);
#7180=ORIENTED_EDGE('',*,*,#5190,.T.);
#7181=ORIENTED_EDGE('',*,*,#5191,.T.);
#7182=ORIENTED_EDGE('',*,*,#5190,.F.);
#7183=ORIENTED_EDGE('',*,*,#5101,.T.);
#7184=ORIENTED_EDGE('',*,*,#5192,.T.);
#7185=ORIENTED_EDGE('',*,*,#5193,.T.);
#7186=ORIENTED_EDGE('',*,*,#5192,.F.);
#7187=ORIENTED_EDGE('',*,*,#5100,.T.);
#7188=ORIENTED_EDGE('',*,*,#5160,.T.);
#7189=ORIENTED_EDGE('',*,*,#5183,.F.);
#7190=ORIENTED_EDGE('',*,*,#5194,.T.);
#7191=ORIENTED_EDGE('',*,*,#5195,.F.);
#7192=ORIENTED_EDGE('',*,*,#5196,.T.);
#7193=ORIENTED_EDGE('',*,*,#5185,.F.);
#7194=ORIENTED_EDGE('',*,*,#5197,.F.);
#7195=ORIENTED_EDGE('',*,*,#5198,.F.);
#7196=ORIENTED_EDGE('',*,*,#5194,.F.);
#7197=ORIENTED_EDGE('',*,*,#5187,.F.);
#7198=ORIENTED_EDGE('',*,*,#5199,.F.);
#7199=ORIENTED_EDGE('',*,*,#5200,.F.);
#7200=ORIENTED_EDGE('',*,*,#5197,.T.);
#7201=ORIENTED_EDGE('',*,*,#5189,.F.);
#7202=ORIENTED_EDGE('',*,*,#5201,.F.);
#7203=ORIENTED_EDGE('',*,*,#5202,.F.);
#7204=ORIENTED_EDGE('',*,*,#5199,.T.);
#7205=ORIENTED_EDGE('',*,*,#5191,.F.);
#7206=ORIENTED_EDGE('',*,*,#5203,.T.);
#7207=ORIENTED_EDGE('',*,*,#5204,.F.);
#7208=ORIENTED_EDGE('',*,*,#5201,.T.);
#7209=ORIENTED_EDGE('',*,*,#5193,.F.);
#7210=ORIENTED_EDGE('',*,*,#5205,.F.);
#7211=ORIENTED_EDGE('',*,*,#5206,.F.);
#7212=ORIENTED_EDGE('',*,*,#5203,.F.);
#7213=ORIENTED_EDGE('',*,*,#5139,.F.);
#7214=ORIENTED_EDGE('',*,*,#5207,.F.);
#7215=ORIENTED_EDGE('',*,*,#5205,.T.);
#7216=ORIENTED_EDGE('',*,*,#5159,.F.);
#7217=ORIENTED_EDGE('',*,*,#5149,.F.);
#7218=ORIENTED_EDGE('',*,*,#5208,.T.);
#7219=ORIENTED_EDGE('',*,*,#5140,.F.);
#7220=ORIENTED_EDGE('',*,*,#5208,.F.);
#7221=ORIENTED_EDGE('',*,*,#5148,.F.);
#7222=ORIENTED_EDGE('',*,*,#5146,.F.);
#7223=ORIENTED_EDGE('',*,*,#5141,.F.);
#7224=ORIENTED_EDGE('',*,*,#5056,.T.);
#7225=ORIENTED_EDGE('',*,*,#5209,.T.);
#7226=ORIENTED_EDGE('',*,*,#5207,.T.);
#7227=ORIENTED_EDGE('',*,*,#5055,.T.);
#7228=ORIENTED_EDGE('',*,*,#5210,.T.);
#7229=ORIENTED_EDGE('',*,*,#5206,.T.);
#7230=ORIENTED_EDGE('',*,*,#5209,.F.);
#7231=ORIENTED_EDGE('',*,*,#5054,.T.);
#7232=ORIENTED_EDGE('',*,*,#5211,.T.);
#7233=ORIENTED_EDGE('',*,*,#5204,.T.);
#7234=ORIENTED_EDGE('',*,*,#5210,.F.);
#7235=ORIENTED_EDGE('',*,*,#5053,.T.);
#7236=ORIENTED_EDGE('',*,*,#5212,.T.);
#7237=ORIENTED_EDGE('',*,*,#5202,.T.);
#7238=ORIENTED_EDGE('',*,*,#5211,.F.);
#7239=ORIENTED_EDGE('',*,*,#5052,.T.);
#7240=ORIENTED_EDGE('',*,*,#5213,.T.);
#7241=ORIENTED_EDGE('',*,*,#5200,.T.);
#7242=ORIENTED_EDGE('',*,*,#5212,.F.);
#7243=ORIENTED_EDGE('',*,*,#5051,.T.);
#7244=ORIENTED_EDGE('',*,*,#5214,.T.);
#7245=ORIENTED_EDGE('',*,*,#5198,.T.);
#7246=ORIENTED_EDGE('',*,*,#5213,.F.);
#7247=ORIENTED_EDGE('',*,*,#5050,.T.);
#7248=ORIENTED_EDGE('',*,*,#5215,.T.);
#7249=ORIENTED_EDGE('',*,*,#5195,.T.);
#7250=ORIENTED_EDGE('',*,*,#5214,.F.);
#7251=ORIENTED_EDGE('',*,*,#5049,.T.);
#7252=ORIENTED_EDGE('',*,*,#5216,.T.);
#7253=ORIENTED_EDGE('',*,*,#5217,.T.);
#7254=ORIENTED_EDGE('',*,*,#5215,.F.);
#7255=ORIENTED_EDGE('',*,*,#5048,.T.);
#7256=ORIENTED_EDGE('',*,*,#5218,.T.);
#7257=ORIENTED_EDGE('',*,*,#5219,.T.);
#7258=ORIENTED_EDGE('',*,*,#5216,.F.);
#7259=ORIENTED_EDGE('',*,*,#5047,.T.);
#7260=ORIENTED_EDGE('',*,*,#5220,.T.);
#7261=ORIENTED_EDGE('',*,*,#5221,.T.);
#7262=ORIENTED_EDGE('',*,*,#5218,.F.);
#7263=ORIENTED_EDGE('',*,*,#5046,.T.);
#7264=ORIENTED_EDGE('',*,*,#5222,.T.);
#7265=ORIENTED_EDGE('',*,*,#5223,.T.);
#7266=ORIENTED_EDGE('',*,*,#5220,.F.);
#7267=ORIENTED_EDGE('',*,*,#5045,.T.);
#7268=ORIENTED_EDGE('',*,*,#5224,.T.);
#7269=ORIENTED_EDGE('',*,*,#5225,.T.);
#7270=ORIENTED_EDGE('',*,*,#5222,.F.);
#7271=ORIENTED_EDGE('',*,*,#5043,.T.);
#7272=ORIENTED_EDGE('',*,*,#5226,.T.);
#7273=ORIENTED_EDGE('',*,*,#5227,.T.);
#7274=ORIENTED_EDGE('',*,*,#5228,.T.);
#7275=ORIENTED_EDGE('',*,*,#5229,.T.);
#7276=ORIENTED_EDGE('',*,*,#5226,.F.);
#7277=ORIENTED_EDGE('',*,*,#5042,.T.);
#7278=ORIENTED_EDGE('',*,*,#5230,.T.);
#7279=ORIENTED_EDGE('',*,*,#5231,.T.);
#7280=ORIENTED_EDGE('',*,*,#5230,.F.);
#7281=ORIENTED_EDGE('',*,*,#5041,.T.);
#7282=ORIENTED_EDGE('',*,*,#5232,.T.);
#7283=ORIENTED_EDGE('',*,*,#5044,.T.);
#7284=ORIENTED_EDGE('',*,*,#5228,.F.);
#7285=ORIENTED_EDGE('',*,*,#5233,.T.);
#7286=ORIENTED_EDGE('',*,*,#5224,.F.);
#7287=ORIENTED_EDGE('',*,*,#5234,.T.);
#7288=ORIENTED_EDGE('',*,*,#5232,.F.);
#7289=ORIENTED_EDGE('',*,*,#5040,.T.);
#7290=ORIENTED_EDGE('',*,*,#5091,.T.);
#7291=ORIENTED_EDGE('',*,*,#5181,.F.);
#7292=ORIENTED_EDGE('',*,*,#5196,.F.);
#7293=ORIENTED_EDGE('',*,*,#5217,.F.);
#7294=ORIENTED_EDGE('',*,*,#5235,.F.);
#7295=ORIENTED_EDGE('',*,*,#5179,.F.);
#7296=ORIENTED_EDGE('',*,*,#5235,.T.);
#7297=ORIENTED_EDGE('',*,*,#5219,.F.);
#7298=ORIENTED_EDGE('',*,*,#5236,.T.);
#7299=ORIENTED_EDGE('',*,*,#5177,.F.);
#7300=ORIENTED_EDGE('',*,*,#5236,.F.);
#7301=ORIENTED_EDGE('',*,*,#5221,.F.);
#7302=ORIENTED_EDGE('',*,*,#5237,.F.);
#7303=ORIENTED_EDGE('',*,*,#5238,.T.);
#7304=ORIENTED_EDGE('',*,*,#5239,.T.);
#7305=ORIENTED_EDGE('',*,*,#5240,.T.);
#7306=ORIENTED_EDGE('',*,*,#5175,.F.);
#7307=ORIENTED_EDGE('',*,*,#5237,.T.);
#7308=ORIENTED_EDGE('',*,*,#5223,.F.);
#7309=ORIENTED_EDGE('',*,*,#5241,.T.);
#7310=ORIENTED_EDGE('',*,*,#5161,.F.);
#7311=ORIENTED_EDGE('',*,*,#5241,.F.);
#7312=ORIENTED_EDGE('',*,*,#5225,.F.);
#7313=ORIENTED_EDGE('',*,*,#5242,.T.);
#7314=ORIENTED_EDGE('',*,*,#5174,.F.);
#7315=ORIENTED_EDGE('',*,*,#5242,.F.);
#7316=ORIENTED_EDGE('',*,*,#5233,.F.);
#7317=ORIENTED_EDGE('',*,*,#5243,.T.);
#7318=ORIENTED_EDGE('',*,*,#5172,.F.);
#7319=ORIENTED_EDGE('',*,*,#5243,.F.);
#7320=ORIENTED_EDGE('',*,*,#5227,.F.);
#7321=ORIENTED_EDGE('',*,*,#5244,.F.);
#7322=ORIENTED_EDGE('',*,*,#5170,.F.);
#7323=ORIENTED_EDGE('',*,*,#5244,.T.);
#7324=ORIENTED_EDGE('',*,*,#5229,.F.);
#7325=ORIENTED_EDGE('',*,*,#5245,.T.);
#7326=ORIENTED_EDGE('',*,*,#5169,.F.);
#7327=ORIENTED_EDGE('',*,*,#5245,.F.);
#7328=ORIENTED_EDGE('',*,*,#5231,.F.);
#7329=ORIENTED_EDGE('',*,*,#5246,.F.);
#7330=ORIENTED_EDGE('',*,*,#5167,.F.);
#7331=ORIENTED_EDGE('',*,*,#5246,.T.);
#7332=ORIENTED_EDGE('',*,*,#5234,.F.);
#7333=ORIENTED_EDGE('',*,*,#5247,.T.);
#7334=ORIENTED_EDGE('',*,*,#5086,.F.);
#7335=ORIENTED_EDGE('',*,*,#5165,.F.);
#7336=ORIENTED_EDGE('',*,*,#5247,.F.);
#7337=ORIENTED_EDGE('',*,*,#5090,.F.);
#7338=ORIENTED_EDGE('',*,*,#5119,.F.);
#7339=ORIENTED_EDGE('',*,*,#5123,.F.);
#7340=ORIENTED_EDGE('',*,*,#5067,.F.);
#7341=ORIENTED_EDGE('',*,*,#5063,.F.);
#7342=ORIENTED_EDGE('',*,*,#5238,.F.);
#7343=ORIENTED_EDGE('',*,*,#5248,.T.);
#7344=ORIENTED_EDGE('',*,*,#5157,.F.);
#7345=ORIENTED_EDGE('',*,*,#5248,.F.);
#7346=ORIENTED_EDGE('',*,*,#5239,.F.);
#7347=ORIENTED_EDGE('',*,*,#5249,.T.);
#7348=ORIENTED_EDGE('',*,*,#5156,.F.);
#7349=ORIENTED_EDGE('',*,*,#5249,.F.);
#7350=ORIENTED_EDGE('',*,*,#5240,.F.);
#7351=ORIENTED_EDGE('',*,*,#5250,.T.);
#7352=ORIENTED_EDGE('',*,*,#5155,.F.);
#7353=ORIENTED_EDGE('',*,*,#5250,.F.);
#7354=ORIENTED_EDGE('',*,*,#5129,.F.);
#7355=ORIENTED_EDGE('',*,*,#5158,.T.);
#7356=ORIENTED_EDGE('',*,*,#5135,.F.);
#7357=ORIENTED_EDGE('',*,*,#5133,.F.);
#8382=PLANE('',#9548);
#8383=PLANE('',#9557);
#8384=PLANE('',#9558);
#8385=PLANE('',#9559);
#8386=PLANE('',#9560);
#8387=PLANE('',#9561);
#8388=PLANE('',#9562);
#8389=PLANE('',#9563);
#8390=PLANE('',#9567);
#8391=PLANE('',#9576);
#8392=PLANE('',#9577);
#8393=PLANE('',#9578);
#8394=PLANE('',#9580);
#8395=PLANE('',#9581);
#8396=PLANE('',#9582);
#8397=PLANE('',#9584);
#8398=PLANE('',#9585);
#8399=PLANE('',#9586);
#8400=PLANE('',#9587);
#8401=PLANE('',#9588);
#8402=PLANE('',#9589);
#8403=PLANE('',#9590);
#8404=PLANE('',#9592);
#8405=PLANE('',#9594);
#8406=PLANE('',#9599);
#8407=PLANE('',#9600);
#8408=PLANE('',#9601);
#8409=PLANE('',#9602);
#8410=PLANE('',#9603);
#8411=PLANE('',#9604);
#8412=PLANE('',#9605);
#8413=PLANE('',#9606);
#8414=PLANE('',#9607);
#8415=PLANE('',#9608);
#8416=PLANE('',#9609);
#8417=PLANE('',#9610);
#8418=PLANE('',#9611);
#8419=PLANE('',#9612);
#8420=PLANE('',#9613);
#8421=PLANE('',#9614);
#8422=PLANE('',#9615);
#8423=PLANE('',#9616);
#8424=PLANE('',#9617);
#8425=PLANE('',#9618);
#8426=PLANE('',#9619);
#8427=PLANE('',#9620);
#8428=PLANE('',#9621);
#8429=PLANE('',#9622);
#8430=PLANE('',#9623);
#8431=PLANE('',#9624);
#8432=PLANE('',#9625);
#8433=PLANE('',#9626);
#8434=PLANE('',#9627);
#8435=PLANE('',#9628);
#8436=PLANE('',#9629);
#8437=PLANE('',#9630);
#8438=PLANE('',#9631);
#8439=PLANE('',#9632);
#8440=PLANE('',#9633);
#8441=PLANE('',#9634);
#8442=PLANE('',#9635);
#8443=PLANE('',#9636);
#8444=PLANE('',#9637);
#8445=PLANE('',#9638);
#8446=PLANE('',#9639);
#8447=PLANE('',#9640);
#8448=PLANE('',#9641);
#8449=PLANE('',#9642);
#8450=PLANE('',#9643);
#8451=PLANE('',#9644);
#8452=PLANE('',#9648);
#8453=PLANE('',#9649);
#8454=PLANE('',#9650);
#8455=PLANE('',#9651);
#8456=PLANE('',#9652);
#8457=PLANE('',#9653);
#8458=PLANE('',#9654);
#8459=PLANE('',#9655);
#8460=PLANE('',#9656);
#8461=PLANE('',#9657);
#8462=PLANE('',#9658);
#8463=PLANE('',#9659);
#8464=PLANE('',#9663);
#8808=ADVANCED_FACE('',(#1087),#408,.F.);
#8809=ADVANCED_FACE('',(#1088,#608,#609),#8382,.F.);
#8810=ADVANCED_FACE('',(#1089),#517,.F.);
#8811=ADVANCED_FACE('',(#1090),#409,.F.);
#8812=ADVANCED_FACE('',(#1091),#518,.F.);
#8813=ADVANCED_FACE('',(#1092),#8383,.T.);
#8814=ADVANCED_FACE('',(#1093),#8384,.T.);
#8815=ADVANCED_FACE('',(#1094),#8385,.T.);
#8816=ADVANCED_FACE('',(#1095),#8386,.T.);
#8817=ADVANCED_FACE('',(#1096),#8387,.T.);
#8818=ADVANCED_FACE('',(#1097),#8388,.T.);
#8819=ADVANCED_FACE('',(#1098),#8389,.T.);
#8820=ADVANCED_FACE('',(#1099),#410,.F.);
#8821=ADVANCED_FACE('',(#1100,#610,#611),#8390,.T.);
#8822=ADVANCED_FACE('',(#1101),#519,.F.);
#8823=ADVANCED_FACE('',(#1102),#411,.F.);
#8824=ADVANCED_FACE('',(#1103),#520,.F.);
#8825=ADVANCED_FACE('',(#1104),#8391,.T.);
#8826=ADVANCED_FACE('',(#1105),#8392,.T.);
#8827=ADVANCED_FACE('',(#1106),#8393,.T.);
#8828=ADVANCED_FACE('',(#1107),#8394,.T.);
#8829=ADVANCED_FACE('',(#1108),#8395,.T.);
#8830=ADVANCED_FACE('',(#1109),#8396,.T.);
#8831=ADVANCED_FACE('',(#1110),#8397,.T.);
#8832=ADVANCED_FACE('',(#1111),#8398,.T.);
#8833=ADVANCED_FACE('',(#1112),#8399,.T.);
#8834=ADVANCED_FACE('',(#1113),#8400,.T.);
#8835=ADVANCED_FACE('',(#1114),#8401,.T.);
#8836=ADVANCED_FACE('',(#1115),#8402,.T.);
#8837=ADVANCED_FACE('',(#1116),#8403,.T.);
#8838=ADVANCED_FACE('',(#1117),#8404,.T.);
#8839=ADVANCED_FACE('',(#1118,#612,#613,#614),#8405,.T.);
#8840=ADVANCED_FACE('',(#1119),#521,.F.);
#8841=ADVANCED_FACE('',(#1120),#8406,.T.);
#8842=ADVANCED_FACE('',(#1121),#8407,.T.);
#8843=ADVANCED_FACE('',(#1122),#8408,.T.);
#8844=ADVANCED_FACE('',(#1123),#8409,.T.);
#8845=ADVANCED_FACE('',(#1124),#8410,.T.);
#8846=ADVANCED_FACE('',(#1125),#8411,.T.);
#8847=ADVANCED_FACE('',(#1126),#8412,.T.);
#8848=ADVANCED_FACE('',(#1127),#8413,.T.);
#8849=ADVANCED_FACE('',(#1128),#8414,.T.);
#8850=ADVANCED_FACE('',(#1129),#8415,.T.);
#8851=ADVANCED_FACE('',(#1130),#8416,.T.);
#8852=ADVANCED_FACE('',(#1131),#8417,.T.);
#8853=ADVANCED_FACE('',(#1132),#8418,.T.);
#8854=ADVANCED_FACE('',(#1133),#8419,.T.);
#8855=ADVANCED_FACE('',(#1134),#8420,.T.);
#8856=ADVANCED_FACE('',(#1135),#8421,.T.);
#8857=ADVANCED_FACE('',(#1136),#8422,.T.);
#8858=ADVANCED_FACE('',(#1137),#8423,.T.);
#8859=ADVANCED_FACE('',(#1138),#8424,.T.);
#8860=ADVANCED_FACE('',(#1139),#8425,.T.);
#8861=ADVANCED_FACE('',(#1140),#8426,.T.);
#8862=ADVANCED_FACE('',(#1141),#8427,.T.);
#8863=ADVANCED_FACE('',(#1142),#8428,.T.);
#8864=ADVANCED_FACE('',(#1143),#8429,.T.);
#8865=ADVANCED_FACE('',(#1144),#8430,.T.);
#8866=ADVANCED_FACE('',(#1145),#8431,.T.);
#8867=ADVANCED_FACE('',(#1146),#8432,.T.);
#8868=ADVANCED_FACE('',(#1147),#8433,.T.);
#8869=ADVANCED_FACE('',(#1148),#8434,.T.);
#8870=ADVANCED_FACE('',(#1149),#8435,.T.);
#8871=ADVANCED_FACE('',(#1150),#8436,.T.);
#8872=ADVANCED_FACE('',(#1151),#8437,.T.);
#8873=ADVANCED_FACE('',(#1152),#8438,.T.);
#8874=ADVANCED_FACE('',(#1153),#8439,.T.);
#8875=ADVANCED_FACE('',(#1154),#8440,.T.);
#8876=ADVANCED_FACE('',(#1155),#8441,.T.);
#8877=ADVANCED_FACE('',(#1156),#8442,.T.);
#8878=ADVANCED_FACE('',(#1157),#8443,.T.);
#8879=ADVANCED_FACE('',(#1158),#8444,.T.);
#8880=ADVANCED_FACE('',(#1159),#8445,.T.);
#8881=ADVANCED_FACE('',(#1160),#8446,.T.);
#8882=ADVANCED_FACE('',(#1161),#8447,.T.);
#8883=ADVANCED_FACE('',(#1162),#8448,.T.);
#8884=ADVANCED_FACE('',(#1163),#8449,.T.);
#8885=ADVANCED_FACE('',(#1164),#8450,.T.);
#8886=ADVANCED_FACE('',(#1165,#615,#616,#617),#8451,.T.);
#8887=ADVANCED_FACE('',(#1166),#8452,.T.);
#8888=ADVANCED_FACE('',(#1167),#8453,.F.);
#8889=ADVANCED_FACE('',(#1168),#8454,.F.);
#8890=ADVANCED_FACE('',(#1169),#8455,.F.);
#8891=ADVANCED_FACE('',(#1170),#8456,.T.);
#8892=ADVANCED_FACE('',(#1171),#8457,.T.);
#8893=ADVANCED_FACE('',(#1172),#8458,.T.);
#8894=ADVANCED_FACE('',(#1173),#8459,.T.);
#8895=ADVANCED_FACE('',(#1174),#8460,.T.);
#8896=ADVANCED_FACE('',(#1175),#8461,.T.);
#8897=ADVANCED_FACE('',(#1176),#8462,.F.);
#8898=ADVANCED_FACE('',(#1177),#8463,.F.);
#8899=ADVANCED_FACE('',(#1178),#522,.F.);
#8900=ADVANCED_FACE('',(#1179),#523,.F.);
#8901=ADVANCED_FACE('',(#1180),#524,.F.);
#8902=ADVANCED_FACE('',(#1181),#8464,.T.);
#9089=CLOSED_SHELL('',(#8808,#8809,#8810,#8811,#8812,#8813,#8814,#8815,
#8816,#8817,#8818,#8819,#8820,#8821,#8822,#8823,#8824,#8825,#8826,#8827,
#8828,#8829,#8830,#8831,#8832,#8833,#8834,#8835,#8836,#8837,#8838,#8839,
#8840,#8841,#8842,#8843,#8844,#8845,#8846,#8847,#8848,#8849,#8850,#8851,
#8852,#8853,#8854,#8855,#8856,#8857,#8858,#8859,#8860,#8861,#8862,#8863,
#8864,#8865,#8866,#8867,#8868,#8869,#8870,#8871,#8872,#8873,#8874,#8875,
#8876,#8877,#8878,#8879,#8880,#8881,#8882,#8883,#8884,#8885,#8886,#8887,
#8888,#8889,#8890,#8891,#8892,#8893,#8894,#8895,#8896,#8897,#8898,#8899,
#8900,#8901,#8902));
#9544=AXIS2_PLACEMENT_3D('',#13996,#10995,#10996);
#9545=AXIS2_PLACEMENT_3D('',#13997,#10997,#10998);
#9546=AXIS2_PLACEMENT_3D('',#13999,#10999,#11000);
#9547=AXIS2_PLACEMENT_3D('',#14002,#11002,#11003);
#9548=AXIS2_PLACEMENT_3D('',#14003,#11004,#11005);
#9549=AXIS2_PLACEMENT_3D('',#14050,#11028,#11029);
#9550=AXIS2_PLACEMENT_3D('',#14053,#11031,#11032);
#9551=AXIS2_PLACEMENT_3D('',#14054,#11033,#11034);
#9552=AXIS2_PLACEMENT_3D('',#14057,#11036,#11037);
#9553=AXIS2_PLACEMENT_3D('',#14058,#11038,#11039);
#9554=AXIS2_PLACEMENT_3D('',#14061,#11041,#11042);
#9555=AXIS2_PLACEMENT_3D('',#14062,#11043,#11044);
#9556=AXIS2_PLACEMENT_3D('',#14065,#11046,#11047);
#9557=AXIS2_PLACEMENT_3D('',#14066,#11048,#11049);
#9558=AXIS2_PLACEMENT_3D('',#14079,#11056,#11057);
#9559=AXIS2_PLACEMENT_3D('',#14085,#11061,#11062);
#9560=AXIS2_PLACEMENT_3D('',#14093,#11067,#11068);
#9561=AXIS2_PLACEMENT_3D('',#14099,#11072,#11073);
#9562=AXIS2_PLACEMENT_3D('',#14107,#11078,#11079);
#9563=AXIS2_PLACEMENT_3D('',#14110,#11082,#11083);
#9564=AXIS2_PLACEMENT_3D('',#14114,#11086,#11087);
#9565=AXIS2_PLACEMENT_3D('',#14116,#11088,#11089);
#9566=AXIS2_PLACEMENT_3D('',#14119,#11091,#11092);
#9567=AXIS2_PLACEMENT_3D('',#14120,#11093,#11094);
#9568=AXIS2_PLACEMENT_3D('',#14124,#11096,#11097);
#9569=AXIS2_PLACEMENT_3D('',#14165,#11118,#11119);
#9570=AXIS2_PLACEMENT_3D('',#14166,#11120,#11121);
#9571=AXIS2_PLACEMENT_3D('',#14169,#11123,#11124);
#9572=AXIS2_PLACEMENT_3D('',#14170,#11125,#11126);
#9573=AXIS2_PLACEMENT_3D('',#14173,#11128,#11129);
#9574=AXIS2_PLACEMENT_3D('',#14174,#11130,#11131);
#9575=AXIS2_PLACEMENT_3D('',#14177,#11133,#11134);
#9576=AXIS2_PLACEMENT_3D('',#14178,#11135,#11136);
#9577=AXIS2_PLACEMENT_3D('',#14184,#11140,#11141);
#9578=AXIS2_PLACEMENT_3D('',#14186,#11143,#11144);
#9579=AXIS2_PLACEMENT_3D('',#14188,#11145,#11146);
#9580=AXIS2_PLACEMENT_3D('',#14190,#11148,#11149);
#9581=AXIS2_PLACEMENT_3D('',#14194,#11152,#11153);
#9582=AXIS2_PLACEMENT_3D('',#14197,#11156,#11157);
#9583=AXIS2_PLACEMENT_3D('',#14199,#11158,#11159);
#9584=AXIS2_PLACEMENT_3D('',#14201,#11161,#11162);
#9585=AXIS2_PLACEMENT_3D('',#14202,#11163,#11164);
#9586=AXIS2_PLACEMENT_3D('',#14208,#11168,#11169);
#9587=AXIS2_PLACEMENT_3D('',#14214,#11173,#11174);
#9588=AXIS2_PLACEMENT_3D('',#14220,#11178,#11179);
#9589=AXIS2_PLACEMENT_3D('',#14223,#11182,#11183);
#9590=AXIS2_PLACEMENT_3D('',#14229,#11187,#11188);
#9591=AXIS2_PLACEMENT_3D('',#14231,#11189,#11190);
#9592=AXIS2_PLACEMENT_3D('',#14233,#11192,#11193);
#9593=AXIS2_PLACEMENT_3D('',#14235,#11194,#11195);
#9594=AXIS2_PLACEMENT_3D('',#14237,#11197,#11198);
#9595=AXIS2_PLACEMENT_3D('',#14240,#11200,#11201);
#9596=AXIS2_PLACEMENT_3D('',#14242,#11202,#11203);
#9597=AXIS2_PLACEMENT_3D('',#14244,#11204,#11205);
#9598=AXIS2_PLACEMENT_3D('',#14245,#11206,#11207);
#9599=AXIS2_PLACEMENT_3D('',#14247,#11209,#11210);
#9600=AXIS2_PLACEMENT_3D('',#14251,#11213,#11214);
#9601=AXIS2_PLACEMENT_3D('',#14257,#11218,#11219);
#9602=AXIS2_PLACEMENT_3D('',#14261,#11222,#11223);
#9603=AXIS2_PLACEMENT_3D('',#14265,#11226,#11227);
#9604=AXIS2_PLACEMENT_3D('',#14269,#11230,#11231);
#9605=AXIS2_PLACEMENT_3D('',#14273,#11234,#11235);
#9606=AXIS2_PLACEMENT_3D('',#14277,#11238,#11239);
#9607=AXIS2_PLACEMENT_3D('',#14279,#11241,#11242);
#9608=AXIS2_PLACEMENT_3D('',#14283,#11245,#11246);
#9609=AXIS2_PLACEMENT_3D('',#14287,#11249,#11250);
#9610=AXIS2_PLACEMENT_3D('',#14291,#11253,#11254);
#9611=AXIS2_PLACEMENT_3D('',#14295,#11257,#11258);
#9612=AXIS2_PLACEMENT_3D('',#14299,#11261,#11262);
#9613=AXIS2_PLACEMENT_3D('',#14303,#11265,#11266);
#9614=AXIS2_PLACEMENT_3D('',#14307,#11269,#11270);
#9615=AXIS2_PLACEMENT_3D('',#14311,#11273,#11274);
#9616=AXIS2_PLACEMENT_3D('',#14315,#11277,#11278);
#9617=AXIS2_PLACEMENT_3D('',#14317,#11280,#11281);
#9618=AXIS2_PLACEMENT_3D('',#14323,#11285,#11286);
#9619=AXIS2_PLACEMENT_3D('',#14327,#11289,#11290);
#9620=AXIS2_PLACEMENT_3D('',#14331,#11293,#11294);
#9621=AXIS2_PLACEMENT_3D('',#14335,#11297,#11298);
#9622=AXIS2_PLACEMENT_3D('',#14339,#11301,#11302);
#9623=AXIS2_PLACEMENT_3D('',#14343,#11305,#11306);
#9624=AXIS2_PLACEMENT_3D('',#14346,#11309,#11310);
#9625=AXIS2_PLACEMENT_3D('',#14347,#11311,#11312);
#9626=AXIS2_PLACEMENT_3D('',#14349,#11314,#11315);
#9627=AXIS2_PLACEMENT_3D('',#14351,#11317,#11318);
#9628=AXIS2_PLACEMENT_3D('',#14353,#11320,#11321);
#9629=AXIS2_PLACEMENT_3D('',#14355,#11323,#11324);
#9630=AXIS2_PLACEMENT_3D('',#14357,#11326,#11327);
#9631=AXIS2_PLACEMENT_3D('',#14359,#11329,#11330);
#9632=AXIS2_PLACEMENT_3D('',#14361,#11332,#11333);
#9633=AXIS2_PLACEMENT_3D('',#14365,#11336,#11337);
#9634=AXIS2_PLACEMENT_3D('',#14369,#11340,#11341);
#9635=AXIS2_PLACEMENT_3D('',#14373,#11344,#11345);
#9636=AXIS2_PLACEMENT_3D('',#14377,#11348,#11349);
#9637=AXIS2_PLACEMENT_3D('',#14381,#11352,#11353);
#9638=AXIS2_PLACEMENT_3D('',#14387,#11357,#11358);
#9639=AXIS2_PLACEMENT_3D('',#14391,#11361,#11362);
#9640=AXIS2_PLACEMENT_3D('',#14395,#11365,#11366);
#9641=AXIS2_PLACEMENT_3D('',#14397,#11368,#11369);
#9642=AXIS2_PLACEMENT_3D('',#14399,#11371,#11372);
#9643=AXIS2_PLACEMENT_3D('',#14401,#11374,#11375);
#9644=AXIS2_PLACEMENT_3D('',#14403,#11377,#11378);
#9645=AXIS2_PLACEMENT_3D('',#14406,#11380,#11381);
#9646=AXIS2_PLACEMENT_3D('',#14408,#11382,#11383);
#9647=AXIS2_PLACEMENT_3D('',#14410,#11384,#11385);
#9648=AXIS2_PLACEMENT_3D('',#14411,#11386,#11387);
#9649=AXIS2_PLACEMENT_3D('',#14413,#11389,#11390);
#9650=AXIS2_PLACEMENT_3D('',#14415,#11392,#11393);
#9651=AXIS2_PLACEMENT_3D('',#14417,#11395,#11396);
#9652=AXIS2_PLACEMENT_3D('',#14419,#11398,#11399);
#9653=AXIS2_PLACEMENT_3D('',#14421,#11401,#11402);
#9654=AXIS2_PLACEMENT_3D('',#14423,#11404,#11405);
#9655=AXIS2_PLACEMENT_3D('',#14425,#11407,#11408);
#9656=AXIS2_PLACEMENT_3D('',#14426,#11409,#11410);
#9657=AXIS2_PLACEMENT_3D('',#14427,#11411,#11412);
#9658=AXIS2_PLACEMENT_3D('',#14428,#11413,#11414);
#9659=AXIS2_PLACEMENT_3D('',#14429,#11415,#11416);
#9660=AXIS2_PLACEMENT_3D('',#14430,#11417,#11418);
#9661=AXIS2_PLACEMENT_3D('',#14432,#11420,#11421);
#9662=AXIS2_PLACEMENT_3D('',#14434,#11423,#11424);
#9663=AXIS2_PLACEMENT_3D('',#14436,#11426,#11427);
#10995=DIRECTION('axis',(0.,0.,1.));
#10996=DIRECTION('refdir',(1.,0.,0.));
#10997=DIRECTION('center_axis',(-1.,0.,0.));
#10998=DIRECTION('ref_axis',(0.,0.,-1.));
#10999=DIRECTION('center_axis',(-1.,0.,0.));
#11000=DIRECTION('ref_axis',(0.,0.,-1.));
#11001=DIRECTION('',(0.707106781186549,-8.65956056235492E-17,-0.707106781186546));
#11002=DIRECTION('center_axis',(1.,0.,0.));
#11003=DIRECTION('ref_axis',(0.,0.,-1.));
#11004=DIRECTION('center_axis',(1.,0.,0.));
#11005=DIRECTION('ref_axis',(0.,0.,-1.));
#11006=DIRECTION('',(0.,-0.707106781186547,-0.707106781186548));
#11007=DIRECTION('',(0.,-0.923879532511285,-0.382683432365095));
#11008=DIRECTION('',(0.,-1.,0.));
#11009=DIRECTION('',(0.,-0.707106781186548,0.707106781186548));
#11010=DIRECTION('',(0.,0.,1.));
#11011=DIRECTION('',(0.,0.707106781186542,0.707106781186553));
#11012=DIRECTION('',(0.,1.,0.));
#11013=DIRECTION('',(0.,0.,1.));
#11014=DIRECTION('',(0.,-1.,0.));
#11015=DIRECTION('',(0.,-0.707106781186553,0.707106781186542));
#11016=DIRECTION('',(0.,0.,1.));
#11017=DIRECTION('',(0.,0.707106781186548,0.707106781186547));
#11018=DIRECTION('',(0.,1.,0.));
#11019=DIRECTION('',(0.,0.70710678118655,-0.707106781186545));
#11020=DIRECTION('',(0.,0.,-1.));
#11021=DIRECTION('',(0.,1.,0.));
#11022=DIRECTION('',(0.,0.,1.));
#11023=DIRECTION('',(0.,0.707106781186546,0.707106781186549));
#11024=DIRECTION('',(0.,1.,0.));
#11025=DIRECTION('',(0.,0.923879532511286,-0.382683432365093));
#11026=DIRECTION('',(0.,0.707106781186548,-0.707106781186548));
#11027=DIRECTION('',(0.,0.,-1.));
#11028=DIRECTION('center_axis',(1.,0.,0.));
#11029=DIRECTION('ref_axis',(0.,0.,-1.));
#11030=DIRECTION('',(0.,0.,-1.));
#11031=DIRECTION('center_axis',(-1.,0.,0.));
#11032=DIRECTION('ref_axis',(0.,0.,-1.));
#11033=DIRECTION('center_axis',(1.,0.,0.));
#11034=DIRECTION('ref_axis',(0.,0.,-1.));
#11035=DIRECTION('',(1.,0.,0.));
#11036=DIRECTION('center_axis',(1.,0.,0.));
#11037=DIRECTION('ref_axis',(0.,0.,-1.));
#11038=DIRECTION('center_axis',(-1.,0.,0.));
#11039=DIRECTION('ref_axis',(0.,0.,-1.));
#11040=DIRECTION('',(0.707106781186549,-8.65956056235492E-17,-0.707106781186546));
#11041=DIRECTION('center_axis',(1.,0.,0.));
#11042=DIRECTION('ref_axis',(0.,0.,-1.));
#11043=DIRECTION('center_axis',(1.,0.,0.));
#11044=DIRECTION('ref_axis',(0.,0.,-1.));
#11045=DIRECTION('',(1.,0.,0.));
#11046=DIRECTION('center_axis',(1.,0.,0.));
#11047=DIRECTION('ref_axis',(0.,0.,-1.));
#11048=DIRECTION('center_axis',(0.,-0.555570233019621,0.831469612302533));
#11049=DIRECTION('ref_axis',(1.,0.,0.));
#11050=DIRECTION('',(-0.191480453955336,0.816084453438868,0.545290198525925));
#11051=DIRECTION('',(-1.,0.,0.));
#11052=DIRECTION('',(-0.19148045395534,-0.816084453438867,-0.545290198525924));
#11053=DIRECTION('',(0.191480453955301,-0.816084453438874,-0.545290198525928));
#11054=DIRECTION('',(1.,0.,0.));
#11055=DIRECTION('',(0.191480453955304,0.816084453438873,0.545290198525928));
#11056=DIRECTION('center_axis',(0.,-0.382683432365095,0.923879532511285));
#11057=DIRECTION('ref_axis',(1.,0.,0.));
#11058=DIRECTION('',(0.,-0.923879532511285,-0.382683432365095));
#11059=DIRECTION('',(1.,0.,0.));
#11060=DIRECTION('',(0.,0.923879532511285,0.382683432365095));
#11061=DIRECTION('center_axis',(0.707106781186551,-0.270598050073101,0.653281482438184));
#11062=DIRECTION('ref_axis',(0.678598344545843,0.,-0.734509555267759));
#11063=DIRECTION('',(-0.700214507282553,-0.396639656760255,0.593613196009116));
#11064=DIRECTION('',(0.,0.923879532511285,0.382683432365095));
#11065=DIRECTION('',(-0.700214507282553,-0.139281325317155,0.700214507282553));
#11066=DIRECTION('',(0.191480453955321,0.962637248139779,0.191480453955329));
#11067=DIRECTION('center_axis',(0.707106781186544,-0.500000000000003,0.500000000000002));
#11068=DIRECTION('ref_axis',(0.57735026918963,0.,-0.816496580927723));
#11069=DIRECTION('',(0.,-0.707106781186547,-0.707106781186548));
#11070=DIRECTION('',(0.653281482438189,0.191341716182535,-0.732537816328744));
#11071=DIRECTION('',(0.,0.707106781186547,0.707106781186548));
#11072=DIRECTION('center_axis',(0.,-0.195090322016134,0.980785280403229));
#11073=DIRECTION('ref_axis',(1.,0.,0.));
#11074=DIRECTION('',(0.191480453955325,-0.962637248139778,-0.191480453955328));
#11075=DIRECTION('',(-0.191480453955328,0.962637248139777,0.191480453955328));
#11076=DIRECTION('',(-1.,0.,0.));
#11077=DIRECTION('',(-0.191480453955332,-0.962637248139776,-0.191480453955328));
#11078=DIRECTION('center_axis',(-0.707106781186543,-0.270598050073104,0.653281482438191));
#11079=DIRECTION('ref_axis',(0.678598344545851,0.,0.734509555267752));
#11080=DIRECTION('',(0.700214507282561,-0.139281325317153,0.700214507282546));
#11081=DIRECTION('',(-0.700214507282555,0.396639656760308,-0.59361319600908));
#11082=DIRECTION('center_axis',(-0.70710678118654,0.,0.707106781186555));
#11083=DIRECTION('ref_axis',(0.707106781186555,0.,0.70710678118654));
#11084=DIRECTION('',(0.,1.,0.));
#11085=DIRECTION('',(0.678598344545856,0.281084637714812,0.678598344545841));
#11086=DIRECTION('center_axis',(1.,0.,0.));
#11087=DIRECTION('ref_axis',(0.,0.,-1.));
#11088=DIRECTION('center_axis',(1.,0.,0.));
#11089=DIRECTION('ref_axis',(0.,0.,-1.));
#11090=DIRECTION('',(-0.707106781186554,8.65956056235486E-17,-0.707106781186541));
#11091=DIRECTION('center_axis',(-1.,0.,0.));
#11092=DIRECTION('ref_axis',(0.,0.,-1.));
#11093=DIRECTION('center_axis',(1.,0.,0.));
#11094=DIRECTION('ref_axis',(0.,0.,-1.));
#11095=DIRECTION('',(0.,0.,1.));
#11096=DIRECTION('center_axis',(-1.,0.,0.));
#11097=DIRECTION('ref_axis',(0.,0.,-1.));
#11098=DIRECTION('',(0.,0.,1.));
#11099=DIRECTION('',(0.,-0.707106781186548,0.707106781186548));
#11100=DIRECTION('',(0.,-0.923879532511286,0.382683432365093));
#11101=DIRECTION('',(0.,-1.,0.));
#11102=DIRECTION('',(0.,-0.707106781186546,-0.707106781186549));
#11103=DIRECTION('',(0.,0.,-1.));
#11104=DIRECTION('',(0.,-1.,0.));
#11105=DIRECTION('',(0.,0.,1.));
#11106=DIRECTION('',(0.,-0.70710678118655,0.707106781186545));
#11107=DIRECTION('',(0.,-1.,0.));
#11108=DIRECTION('',(0.,-0.707106781186548,-0.707106781186547));
#11109=DIRECTION('',(0.,0.,-1.));
#11110=DIRECTION('',(0.,0.707106781186553,-0.707106781186542));
#11111=DIRECTION('',(0.,1.,0.));
#11112=DIRECTION('',(0.,0.,-1.));
#11113=DIRECTION('',(0.,-1.,0.));
#11114=DIRECTION('',(0.,-0.707106781186542,-0.707106781186553));
#11115=DIRECTION('',(0.,0.,-1.));
#11116=DIRECTION('',(0.,0.707106781186548,-0.707106781186548));
#11117=DIRECTION('',(0.,1.,0.));
#11118=DIRECTION('center_axis',(1.,0.,0.));
#11119=DIRECTION('ref_axis',(0.,0.,-1.));
#11120=DIRECTION('center_axis',(-1.,0.,0.));
#11121=DIRECTION('ref_axis',(0.,0.,-1.));
#11122=DIRECTION('',(-1.,0.,0.));
#11123=DIRECTION('center_axis',(-1.,0.,0.));
#11124=DIRECTION('ref_axis',(0.,0.,-1.));
#11125=DIRECTION('center_axis',(1.,0.,0.));
#11126=DIRECTION('ref_axis',(0.,0.,-1.));
#11127=DIRECTION('',(-0.707106781186554,8.65956056235486E-17,-0.707106781186541));
#11128=DIRECTION('center_axis',(-1.,0.,0.));
#11129=DIRECTION('ref_axis',(0.,0.,-1.));
#11130=DIRECTION('center_axis',(-1.,0.,0.));
#11131=DIRECTION('ref_axis',(0.,0.,-1.));
#11132=DIRECTION('',(-1.,0.,0.));
#11133=DIRECTION('center_axis',(-1.,0.,0.));
#11134=DIRECTION('ref_axis',(0.,0.,-1.));
#11135=DIRECTION('center_axis',(-0.57330218625602,-0.756975158957756,0.313549377219837));
#11136=DIRECTION('ref_axis',(0.479841491130337,0.,0.877355197961359));
#11137=DIRECTION('',(0.,-0.382683432365094,-0.923879532511285));
#11138=DIRECTION('',(0.653281482438184,-0.191341716182538,0.732537816328748));
#11139=DIRECTION('',(-0.653281482438192,0.653281482438192,0.382683432365078));
#11140=DIRECTION('center_axis',(-0.707106781186549,-0.499999999999999,0.499999999999999));
#11141=DIRECTION('ref_axis',(0.577350269189624,0.,0.816496580927727));
#11142=DIRECTION('',(0.,0.707106781186547,0.707106781186548));
#11143=DIRECTION('center_axis',(-0.707106781186547,-0.707106781186548,0.));
#11144=DIRECTION('ref_axis',(0.,0.,1.));
#11145=DIRECTION('center_axis',(0.707106781186547,0.707106781186548,0.));
#11146=DIRECTION('ref_axis',(-0.707106781186548,0.707106781186547,0.));
#11147=DIRECTION('',(0.,0.,1.));
#11148=DIRECTION('center_axis',(0.573302186256015,-0.75697515895776,0.313549377219838));
#11149=DIRECTION('ref_axis',(0.479841491130341,0.,-0.877355197961356));
#11150=DIRECTION('',(0.,0.382683432365094,0.923879532511285));
#11151=DIRECTION('',(-0.653281482438197,-0.653281482438188,-0.382683432365075));
#11152=DIRECTION('center_axis',(0.,-0.923879532511285,0.382683432365094));
#11153=DIRECTION('ref_axis',(0.,-0.382683432365094,-0.923879532511285));
#11154=DIRECTION('',(-1.,0.,0.));
#11155=DIRECTION('',(1.,0.,0.));
#11156=DIRECTION('center_axis',(0.707106781186542,-0.707106781186553,0.));
#11157=DIRECTION('ref_axis',(0.,0.,-1.));
#11158=DIRECTION('center_axis',(-0.707106781186542,0.707106781186553,0.));
#11159=DIRECTION('ref_axis',(0.707106781186553,0.707106781186542,0.));
#11160=DIRECTION('',(0.,0.,-1.));
#11161=DIRECTION('center_axis',(0.,-0.707106781186548,0.707106781186547));
#11162=DIRECTION('ref_axis',(0.,-0.707106781186547,-0.707106781186548));
#11163=DIRECTION('center_axis',(-0.573302186256016,-0.756975158957761,-0.313549377219833));
#11164=DIRECTION('ref_axis',(-0.479841491130335,0.,0.87735519796136));
#11165=DIRECTION('',(0.653281482438192,-0.653281482438192,0.382683432365078));
#11166=DIRECTION('',(-0.653281482438188,0.191341716182541,0.732537816328743));
#11167=DIRECTION('',(0.,0.382683432365089,-0.923879532511287));
#11168=DIRECTION('center_axis',(-0.707106781186547,-0.5,-0.5));
#11169=DIRECTION('ref_axis',(-0.577350269189626,0.,0.816496580927726));
#11170=DIRECTION('',(0.357406744336591,-0.862856209461017,0.357406744336596));
#11171=DIRECTION('',(0.,-0.707106781186548,0.707106781186548));
#11172=DIRECTION('',(0.700214507282551,-0.396639656760267,-0.593613196009111));
#11173=DIRECTION('center_axis',(0.573302186256013,-0.756975158957763,-0.313549377219834));
#11174=DIRECTION('ref_axis',(-0.479841491130337,0.,-0.877355197961358));
#11175=DIRECTION('',(0.653281482438194,0.653281482438185,-0.382683432365085));
#11176=DIRECTION('',(0.,-0.382683432365089,0.923879532511287));
#11177=DIRECTION('',(-0.653281482438194,-0.191341716182545,-0.732537816328737));
#11178=DIRECTION('center_axis',(0.,-0.923879532511287,-0.382683432365089));
#11179=DIRECTION('ref_axis',(0.,0.382683432365089,-0.923879532511287));
#11180=DIRECTION('',(-1.,0.,0.));
#11181=DIRECTION('',(1.,0.,0.));
#11182=DIRECTION('center_axis',(0.707106781186542,-0.500000000000004,-0.500000000000004));
#11183=DIRECTION('ref_axis',(-0.577350269189631,0.,-0.816496580927722));
#11184=DIRECTION('',(0.70021450728255,0.396639656760214,0.593613196009148));
#11185=DIRECTION('',(0.,0.707106781186548,-0.707106781186548));
#11186=DIRECTION('',(0.357406744336595,0.862856209461015,-0.357406744336596));
#11187=DIRECTION('center_axis',(0.707106781186542,-0.707106781186553,0.));
#11188=DIRECTION('ref_axis',(0.,0.,-1.));
#11189=DIRECTION('center_axis',(-0.707106781186542,0.707106781186553,0.));
#11190=DIRECTION('ref_axis',(0.707106781186553,0.707106781186542,0.));
#11191=DIRECTION('',(0.,0.,-1.));
#11192=DIRECTION('center_axis',(-0.707106781186547,-0.707106781186548,0.));
#11193=DIRECTION('ref_axis',(0.,0.,1.));
#11194=DIRECTION('center_axis',(0.707106781186547,0.707106781186548,0.));
#11195=DIRECTION('ref_axis',(-0.707106781186548,0.707106781186547,0.));
#11196=DIRECTION('',(0.,0.,1.));
#11197=DIRECTION('center_axis',(0.,-1.,0.));
#11198=DIRECTION('ref_axis',(0.,0.,-1.));
#11199=DIRECTION('',(-1.,0.,0.));
#11200=DIRECTION('center_axis',(0.,1.,0.));
#11201=DIRECTION('ref_axis',(1.,0.,0.));
#11202=DIRECTION('center_axis',(0.,1.,0.));
#11203=DIRECTION('ref_axis',(1.,0.,0.));
#11204=DIRECTION('center_axis',(0.,1.,0.));
#11205=DIRECTION('ref_axis',(1.,0.,0.));
#11206=DIRECTION('center_axis',(1.,0.,0.));
#11207=DIRECTION('ref_axis',(0.,0.,-1.));
#11208=DIRECTION('',(1.,0.,0.));
#11209=DIRECTION('center_axis',(0.707106781186559,-0.270598050073096,-0.653281482438177));
#11210=DIRECTION('ref_axis',(-0.678598344545835,0.,-0.734509555267767));
#11211=DIRECTION('',(0.,0.923879532511286,-0.382683432365093));
#11212=DIRECTION('',(-0.700214507282542,-0.139281325317168,-0.700214507282561));
#11213=DIRECTION('center_axis',(0.707106781186555,0.,0.70710678118654));
#11214=DIRECTION('ref_axis',(0.70710678118654,0.,-0.707106781186555));
#11215=DIRECTION('',(0.,-1.,0.));
#11216=DIRECTION('',(0.577350269189617,-0.57735026918963,-0.57735026918963));
#11217=DIRECTION('',(-0.678598344545838,0.281084637714811,0.67859834454586));
#11218=DIRECTION('center_axis',(0.707106781186548,0.,0.707106781186548));
#11219=DIRECTION('ref_axis',(0.707106781186548,0.,-0.707106781186548));
#11220=DIRECTION('',(-0.678598344545848,0.281084637714815,0.678598344545848));
#11221=DIRECTION('',(0.,-1.,0.));
#11222=DIRECTION('center_axis',(0.70710678118654,0.500000000000005,0.500000000000005));
#11223=DIRECTION('ref_axis',(0.577350269189634,0.,-0.81649658092772));
#11224=DIRECTION('',(-0.678598344545841,0.678598344545856,0.281084637714812));
#11225=DIRECTION('',(0.,-0.707106781186548,0.707106781186548));
#11226=DIRECTION('center_axis',(0.707106781186555,0.70710678118654,0.));
#11227=DIRECTION('ref_axis',(0.,0.,-1.));
#11228=DIRECTION('',(-0.678598344545839,0.678598344545846,-0.281084637714841));
#11229=DIRECTION('',(0.,0.,1.));
#11230=DIRECTION('center_axis',(0.707106781186559,0.499999999999995,-0.499999999999988));
#11231=DIRECTION('ref_axis',(-0.57735026918961,0.,-0.816496580927737));
#11232=DIRECTION('',(0.,0.707106781186542,0.707106781186553));
#11233=DIRECTION('',(-0.678598344545837,0.281084637714833,-0.678598344545852));
#11234=DIRECTION('center_axis',(0.707106781186555,0.,-0.70710678118654));
#11235=DIRECTION('ref_axis',(-0.70710678118654,0.,-0.707106781186555));
#11236=DIRECTION('',(0.,1.,0.));
#11237=DIRECTION('',(-0.577350269189617,0.57735026918963,-0.57735026918963));
#11238=DIRECTION('center_axis',(0.707106781186555,0.70710678118654,0.));
#11239=DIRECTION('ref_axis',(0.,0.,-1.));
#11240=DIRECTION('',(0.,0.,1.));
#11241=DIRECTION('center_axis',(0.707106781186554,0.499999999999992,0.499999999999999));
#11242=DIRECTION('ref_axis',(0.577350269189622,0.,-0.816496580927729));
#11243=DIRECTION('',(0.,-0.707106781186553,0.707106781186542));
#11244=DIRECTION('',(-0.67859834454584,0.678598344545855,0.281084637714819));
#11245=DIRECTION('center_axis',(0.707106781186555,0.70710678118654,0.));
#11246=DIRECTION('ref_axis',(0.,0.,-1.));
#11247=DIRECTION('',(0.,0.,1.));
#11248=DIRECTION('',(-0.678598344545827,0.678598344545842,-0.281084637714881));
#11249=DIRECTION('center_axis',(0.707106781186577,0.499999999999979,-0.49999999999998));
#11250=DIRECTION('ref_axis',(-0.577350269189594,0.,-0.816496580927748));
#11251=DIRECTION('',(0.,0.707106781186548,0.707106781186547));
#11252=DIRECTION('',(-0.678598344545828,0.281084637714875,-0.678598344545843));
#11253=DIRECTION('center_axis',(0.707106781186555,0.,-0.70710678118654));
#11254=DIRECTION('ref_axis',(-0.70710678118654,0.,-0.707106781186555));
#11255=DIRECTION('',(0.,1.,0.));
#11256=DIRECTION('',(-0.67859834454584,-0.281084637714819,-0.678598344545855));
#11257=DIRECTION('center_axis',(0.707106781186555,-0.499999999999993,-0.499999999999997));
#11258=DIRECTION('ref_axis',(-0.577350269189619,0.,-0.816496580927731));
#11259=DIRECTION('',(0.,0.70710678118655,-0.707106781186545));
#11260=DIRECTION('',(-0.678598344545838,-0.678598344545853,-0.281084637714827));
#11261=DIRECTION('center_axis',(0.707106781186555,-0.70710678118654,0.));
#11262=DIRECTION('ref_axis',(0.,0.,-1.));
#11263=DIRECTION('',(0.,0.,-1.));
#11264=DIRECTION('',(-0.577350269189617,-0.57735026918963,-0.57735026918963));
#11265=DIRECTION('center_axis',(0.707106781186555,0.,-0.70710678118654));
#11266=DIRECTION('ref_axis',(-0.70710678118654,0.,-0.707106781186555));
#11267=DIRECTION('',(0.,1.,0.));
#11268=DIRECTION('',(-0.577350269189617,0.57735026918963,-0.57735026918963));
#11269=DIRECTION('center_axis',(0.707106781186555,0.70710678118654,0.));
#11270=DIRECTION('ref_axis',(0.,0.,-1.));
#11271=DIRECTION('',(0.,0.,1.));
#11272=DIRECTION('',(-0.678598344545838,0.678598344545853,-0.281084637714826));
#11273=DIRECTION('center_axis',(0.707106781186555,0.499999999999996,-0.499999999999993));
#11274=DIRECTION('ref_axis',(-0.577350269189616,0.,-0.816496580927733));
#11275=DIRECTION('',(0.,0.707106781186546,0.707106781186549));
#11276=DIRECTION('',(-0.678598344545837,0.281084637714826,-0.678598344545855));
#11277=DIRECTION('center_axis',(0.707106781186557,0.,-0.707106781186538));
#11278=DIRECTION('ref_axis',(-0.707106781186538,0.,-0.707106781186557));
#11279=DIRECTION('',(0.,1.,0.));
#11280=DIRECTION('center_axis',(0.,-0.707106781186545,-0.70710678118655));
#11281=DIRECTION('ref_axis',(-1.,0.,0.));
#11282=DIRECTION('',(-1.,0.,0.));
#11283=DIRECTION('',(0.,-0.70710678118655,0.707106781186545));
#11284=DIRECTION('',(1.,0.,0.));
#11285=DIRECTION('center_axis',(0.,-1.,0.));
#11286=DIRECTION('ref_axis',(0.,0.,-1.));
#11287=DIRECTION('',(1.,0.,0.));
#11288=DIRECTION('',(0.,0.,1.));
#11289=DIRECTION('center_axis',(0.,0.,-1.));
#11290=DIRECTION('ref_axis',(0.,1.,0.));
#11291=DIRECTION('',(1.,0.,0.));
#11292=DIRECTION('',(0.,-1.,0.));
#11293=DIRECTION('center_axis',(0.,1.,0.));
#11294=DIRECTION('ref_axis',(0.,0.,1.));
#11295=DIRECTION('',(1.,0.,0.));
#11296=DIRECTION('',(0.,0.,-1.));
#11297=DIRECTION('center_axis',(0.,0.707106781186549,-0.707106781186546));
#11298=DIRECTION('ref_axis',(-1.,0.,0.));
#11299=DIRECTION('',(-1.,0.,0.));
#11300=DIRECTION('',(0.,-0.707106781186546,-0.707106781186549));
#11301=DIRECTION('center_axis',(0.,0.,-1.));
#11302=DIRECTION('ref_axis',(0.,1.,0.));
#11303=DIRECTION('',(1.,0.,0.));
#11304=DIRECTION('',(0.,-1.,0.));
#11305=DIRECTION('center_axis',(0.,-0.382683432365093,-0.923879532511286));
#11306=DIRECTION('ref_axis',(-1.,0.,0.));
#11307=DIRECTION('',(0.,-0.923879532511286,0.382683432365093));
#11308=DIRECTION('',(-1.,0.,0.));
#11309=DIRECTION('center_axis',(0.,-0.707106781186548,-0.707106781186548));
#11310=DIRECTION('ref_axis',(0.,0.707106781186548,-0.707106781186548));
#11311=DIRECTION('center_axis',(-0.707106781186551,-0.270598050073099,-0.653281482438184));
#11312=DIRECTION('ref_axis',(-0.678598344545843,0.,0.73450955526776));
#11313=DIRECTION('',(0.70021450728255,-0.13928132531717,-0.700214507282553));
#11314=DIRECTION('center_axis',(-0.707106781186549,0.,-0.707106781186546));
#11315=DIRECTION('ref_axis',(-0.707106781186546,0.,0.707106781186549));
#11316=DIRECTION('',(0.678598344545846,0.281084637714823,-0.678598344545847));
#11317=DIRECTION('center_axis',(-0.707106781186548,0.500000000000001,-0.499999999999999));
#11318=DIRECTION('ref_axis',(-0.577350269189625,0.,0.816496580927727));
#11319=DIRECTION('',(0.678598344545846,0.678598344545847,-0.281084637714823));
#11320=DIRECTION('center_axis',(-0.707106781186548,0.707106781186547,0.));
#11321=DIRECTION('ref_axis',(0.,0.,1.));
#11322=DIRECTION('',(0.577350269189626,0.577350269189626,-0.577350269189626));
#11323=DIRECTION('center_axis',(-0.707106781186548,0.,-0.707106781186547));
#11324=DIRECTION('ref_axis',(-0.707106781186547,0.,0.707106781186548));
#11325=DIRECTION('',(0.577350269189626,-0.577350269189626,-0.577350269189626));
#11326=DIRECTION('center_axis',(-0.707106781186548,-0.707106781186547,0.));
#11327=DIRECTION('ref_axis',(0.,0.,1.));
#11328=DIRECTION('',(0.678598344545847,-0.678598344545847,-0.281084637714821));
#11329=DIRECTION('center_axis',(-0.707106781186548,-0.499999999999998,-0.500000000000002));
#11330=DIRECTION('ref_axis',(-0.577350269189627,0.,0.816496580927725));
#11331=DIRECTION('',(0.678598344545848,-0.281084637714816,-0.678598344545848));
#11332=DIRECTION('center_axis',(-0.707106781186548,0.,-0.707106781186547));
#11333=DIRECTION('ref_axis',(-0.707106781186547,0.,0.707106781186548));
#11334=DIRECTION('',(0.678598344545835,0.281084637714872,-0.678598344545838));
#11335=DIRECTION('',(0.,-1.,0.));
#11336=DIRECTION('center_axis',(-0.707106781186569,0.499999999999984,-0.499999999999985));
#11337=DIRECTION('ref_axis',(-0.577350269189602,0.,0.816496580927743));
#11338=DIRECTION('',(0.678598344545836,0.678598344545836,-0.281084637714873));
#11339=DIRECTION('',(0.,-0.707106781186548,-0.707106781186547));
#11340=DIRECTION('center_axis',(-0.707106781186548,0.707106781186547,0.));
#11341=DIRECTION('ref_axis',(0.,0.,1.));
#11342=DIRECTION('',(0.678598344545846,0.678598344545847,0.281084637714823));
#11343=DIRECTION('',(0.,0.,-1.));
#11344=DIRECTION('center_axis',(-0.707106781186546,0.499999999999997,0.500000000000005));
#11345=DIRECTION('ref_axis',(0.57735026918963,0.,0.816496580927723));
#11346=DIRECTION('',(0.678598344545848,0.281084637714816,0.678598344545848));
#11347=DIRECTION('',(0.,0.707106781186553,-0.707106781186542));
#11348=DIRECTION('center_axis',(-0.707106781186548,0.,0.707106781186547));
#11349=DIRECTION('ref_axis',(0.707106781186547,0.,0.707106781186548));
#11350=DIRECTION('',(0.577350269189626,0.577350269189626,0.577350269189626));
#11351=DIRECTION('',(0.,1.,0.));
#11352=DIRECTION('center_axis',(-0.707106781186548,0.,-0.707106781186547));
#11353=DIRECTION('ref_axis',(-0.707106781186547,0.,0.707106781186548));
#11354=DIRECTION('',(0.678598344545845,0.28108463771483,-0.678598344545845));
#11355=DIRECTION('',(0.,-1.,0.));
#11356=DIRECTION('',(-0.577350269189626,-0.577350269189626,0.577350269189626));
#11357=DIRECTION('center_axis',(-0.707106781186552,0.500000000000001,-0.499999999999993));
#11358=DIRECTION('ref_axis',(-0.577350269189618,0.,0.816496580927731));
#11359=DIRECTION('',(0.,-0.707106781186542,-0.707106781186553));
#11360=DIRECTION('',(0.678598344545846,0.678598344545847,-0.281084637714823));
#11361=DIRECTION('center_axis',(-0.707106781186548,0.707106781186547,0.));
#11362=DIRECTION('ref_axis',(0.,0.,1.));
#11363=DIRECTION('',(0.,0.,-1.));
#11364=DIRECTION('',(0.678598344545853,0.678598344545845,0.281084637714811));
#11365=DIRECTION('center_axis',(-0.707106781186548,0.707106781186547,0.));
#11366=DIRECTION('ref_axis',(0.,0.,1.));
#11367=DIRECTION('',(0.,0.,-1.));
#11368=DIRECTION('center_axis',(-0.707106781186532,0.500000000000011,0.500000000000011));
#11369=DIRECTION('ref_axis',(0.577350269189642,0.,0.816496580927714));
#11370=DIRECTION('',(0.,0.707106781186548,-0.707106781186548));
#11371=DIRECTION('center_axis',(0.,0.,-1.));
#11372=DIRECTION('ref_axis',(0.,1.,0.));
#11373=DIRECTION('',(-1.,0.,0.));
#11374=DIRECTION('center_axis',(0.,0.707106781186547,-0.707106781186548));
#11375=DIRECTION('ref_axis',(-1.,0.,0.));
#11376=DIRECTION('',(1.,0.,0.));
#11377=DIRECTION('center_axis',(0.,1.,0.));
#11378=DIRECTION('ref_axis',(0.,0.,1.));
#11379=DIRECTION('',(-1.,0.,0.));
#11380=DIRECTION('center_axis',(0.,-1.,0.));
#11381=DIRECTION('ref_axis',(1.,0.,0.));
#11382=DIRECTION('center_axis',(0.,-1.,0.));
#11383=DIRECTION('ref_axis',(1.,0.,0.));
#11384=DIRECTION('center_axis',(0.,-1.,0.));
#11385=DIRECTION('ref_axis',(1.,0.,0.));
#11386=DIRECTION('center_axis',(0.,0.707106781186542,0.707106781186553));
#11387=DIRECTION('ref_axis',(1.,0.,0.));
#11388=DIRECTION('',(1.,0.,0.));
#11389=DIRECTION('center_axis',(0.,0.,-1.));
#11390=DIRECTION('ref_axis',(0.,1.,0.));
#11391=DIRECTION('',(1.,0.,0.));
#11392=DIRECTION('center_axis',(0.,-1.,0.));
#11393=DIRECTION('ref_axis',(0.,0.,-1.));
#11394=DIRECTION('',(1.,0.,0.));
#11395=DIRECTION('center_axis',(0.,0.,1.));
#11396=DIRECTION('ref_axis',(0.,-1.,0.));
#11397=DIRECTION('',(-1.,0.,0.));
#11398=DIRECTION('center_axis',(0.,0.707106781186553,-0.707106781186542));
#11399=DIRECTION('ref_axis',(-1.,0.,0.));
#11400=DIRECTION('',(1.,0.,0.));
#11401=DIRECTION('center_axis',(0.,1.,0.));
#11402=DIRECTION('ref_axis',(0.,0.,1.));
#11403=DIRECTION('',(-1.,0.,0.));
#11404=DIRECTION('center_axis',(0.,0.707106781186548,0.707106781186548));
#11405=DIRECTION('ref_axis',(1.,0.,0.));
#11406=DIRECTION('',(1.,0.,0.));
#11407=DIRECTION('center_axis',(0.,0.,1.));
#11408=DIRECTION('ref_axis',(0.,-1.,0.));
#11409=DIRECTION('center_axis',(1.,0.,0.));
#11410=DIRECTION('ref_axis',(0.,0.,-1.));
#11411=DIRECTION('center_axis',(1.,0.,0.));
#11412=DIRECTION('ref_axis',(0.,0.,-1.));
#11413=DIRECTION('center_axis',(1.,0.,0.));
#11414=DIRECTION('ref_axis',(0.,0.,-1.));
#11415=DIRECTION('center_axis',(1.,0.,0.));
#11416=DIRECTION('ref_axis',(0.,0.,-1.));
#11417=DIRECTION('center_axis',(0.,-1.,0.));
#11418=DIRECTION('ref_axis',(1.,0.,0.));
#11419=DIRECTION('',(0.,-1.,0.));
#11420=DIRECTION('center_axis',(0.,-1.,0.));
#11421=DIRECTION('ref_axis',(1.,0.,0.));
#11422=DIRECTION('',(0.,-1.,0.));
#11423=DIRECTION('center_axis',(0.,-1.,0.));
#11424=DIRECTION('ref_axis',(1.,0.,0.));
#11425=DIRECTION('',(0.,-1.,0.));
#11426=DIRECTION('center_axis',(0.,-1.,0.));
#11427=DIRECTION('ref_axis',(0.,0.,-1.));
#13996=CARTESIAN_POINT('',(0.,0.,0.));
#13997=CARTESIAN_POINT('Origin',(0.25,25.,66.5));
#13998=CARTESIAN_POINT('',(0.,25.,68.55));
#13999=CARTESIAN_POINT('Origin',(0.,25.,66.5));
#14000=CARTESIAN_POINT('',(0.5,25.,68.05));
#14001=CARTESIAN_POINT('',(0.25,25.,68.3));
#14002=CARTESIAN_POINT('Origin',(0.5,25.,66.5));
#14003=CARTESIAN_POINT('Origin',(0.,19.075,47.5));
#14004=CARTESIAN_POINT('',(0.,26.3437390864656,94.3366323052791));
#14005=CARTESIAN_POINT('',(0.,3.65,71.6428932188134));
#14006=CARTESIAN_POINT('',(0.,12.9723033905933,80.9651966094067));
#14007=CARTESIAN_POINT('',(0.,26.9795649469519,94.6));
#14008=CARTESIAN_POINT('',(0.,15.0605866884815,89.6629975557115));
#14009=CARTESIAN_POINT('',(0.,34.2343145750508,94.6));
#14010=CARTESIAN_POINT('',(0.,27.0375,94.6));
#14011=CARTESIAN_POINT('',(0.,34.6,94.2343145750508));
#14012=CARTESIAN_POINT('',(0.,42.3109072875254,86.5234072875254));
#14013=CARTESIAN_POINT('',(0.,34.6,73.3656854249492));
#14014=CARTESIAN_POINT('',(0.,34.6,23.75));
#14015=CARTESIAN_POINT('',(0.,34.5343145750508,73.3));
#14016=CARTESIAN_POINT('',(0.,24.2359072875254,63.0015927124745));
#14017=CARTESIAN_POINT('',(0.,34.1,73.3));
#14018=CARTESIAN_POINT('',(0.,27.5375,73.3));
#14019=CARTESIAN_POINT('',(0.,34.1,21.8));
#14020=CARTESIAN_POINT('',(0.,34.1,60.2));
#14021=CARTESIAN_POINT('',(0.,34.5343145750508,21.8));
#14022=CARTESIAN_POINT('',(0.,26.7875,21.8));
#14023=CARTESIAN_POINT('',(0.,34.6,21.7343145750508));
#14024=CARTESIAN_POINT('',(0.,24.2609072875253,32.0734072875253));
#14025=CARTESIAN_POINT('',(0.,34.6,0.765685424949272));
#14026=CARTESIAN_POINT('',(0.,34.6,23.75));
#14027=CARTESIAN_POINT('',(0.,34.2343145750507,0.399999999999999));
#14028=CARTESIAN_POINT('',(0.,42.3109072875254,8.47659271247462));
#14029=CARTESIAN_POINT('',(0.,29.1656854249492,0.4));
#14030=CARTESIAN_POINT('',(0.,23.7375,0.4));
#14031=CARTESIAN_POINT('',(0.,28.8,0.765685424949238));
#14032=CARTESIAN_POINT('',(0.,14.7765927124746,14.7890927124745));
#14033=CARTESIAN_POINT('',(0.,28.8,9.9));
#14034=CARTESIAN_POINT('',(0.,28.8,28.5));
#14035=CARTESIAN_POINT('',(0.,22.2,9.9));
#14036=CARTESIAN_POINT('',(0.,20.8375,9.9));
#14037=CARTESIAN_POINT('',(0.,22.2,4.76568542494924));
#14038=CARTESIAN_POINT('',(0.,22.2,25.9));
#14039=CARTESIAN_POINT('',(0.,22.1343145750508,4.7));
#14040=CARTESIAN_POINT('',(0.,32.0859072875254,14.6515927124747));
#14041=CARTESIAN_POINT('',(0.,13.4795649469519,4.7));
#14042=CARTESIAN_POINT('',(0.,16.0875,4.7));
#14043=CARTESIAN_POINT('',(0.,13.3558711208215,4.751235660365));
#14044=CARTESIAN_POINT('',(0.,8.21024487335069,6.88262383897043));
#14045=CARTESIAN_POINT('',(0.,3.65,14.4571067811865));
#14046=CARTESIAN_POINT('',(0.,-0.827696609406725,18.9348033905933));
#14047=CARTESIAN_POINT('',(0.,3.65,33.9841759407722));
#14048=CARTESIAN_POINT('',(0.,3.65,59.675));
#14049=CARTESIAN_POINT('',(0.,3.65,61.0158240592278));
#14050=CARTESIAN_POINT('Origin',(0.,0.,47.5));
#14051=CARTESIAN_POINT('',(0.,3.65,59.675));
#14052=CARTESIAN_POINT('',(0.,25.,28.55));
#14053=CARTESIAN_POINT('Origin',(0.,25.,26.5));
#14054=CARTESIAN_POINT('Origin',(0.,25.,66.5));
#14055=CARTESIAN_POINT('',(8.,25.,68.05));
#14056=CARTESIAN_POINT('',(0.,25.,68.05));
#14057=CARTESIAN_POINT('Origin',(8.,25.,66.5));
#14058=CARTESIAN_POINT('Origin',(0.25,25.,26.5));
#14059=CARTESIAN_POINT('',(0.5,25.,28.05));
#14060=CARTESIAN_POINT('',(0.25,25.,28.3));
#14061=CARTESIAN_POINT('Origin',(0.5,25.,26.5));
#14062=CARTESIAN_POINT('Origin',(0.,25.,26.5));
#14063=CARTESIAN_POINT('',(8.,25.,28.05));
#14064=CARTESIAN_POINT('',(0.,25.,28.05));
#14065=CARTESIAN_POINT('Origin',(8.,25.,26.5));
#14066=CARTESIAN_POINT('Origin',(0.,25.9299291191192,94.4946300940827));
#14067=CARTESIAN_POINT('',(99.6456708580913,26.1430277504891,94.6370180473338));
#14068=CARTESIAN_POINT('',(99.6,26.3376756975437,94.7670776474706));
#14069=CARTESIAN_POINT('',(98.9677437265672,29.0323346284133,96.5675911815562));
#14070=CARTESIAN_POINT('',(0.4,26.3376756975437,94.7670776474706));
#14071=CARTESIAN_POINT('',(0.,26.3376756975437,94.7670776474706));
#14072=CARTESIAN_POINT('',(0.354329141908731,26.143027750489,94.6370180473338));
#14073=CARTESIAN_POINT('',(-0.800981938914284,21.2191235478949,91.3469704439993));
#14074=CARTESIAN_POINT('',(0.5,25.5221825406948,94.2221825406948));
#14075=CARTESIAN_POINT('',(2.11739775967216,18.6288775613602,89.6162234088404));
#14076=CARTESIAN_POINT('',(99.5,25.5221825406948,94.2221825406948));
#14077=CARTESIAN_POINT('',(0.,25.5221825406948,94.2221825406948));
#14078=CARTESIAN_POINT('',(96.0493640279813,10.8156664808431,84.3956026712843));
#14079=CARTESIAN_POINT('Origin',(0.,26.387867965644,94.787867965644));
#14080=CARTESIAN_POINT('',(99.6,26.4380602337443,94.8086582838175));
#14081=CARTESIAN_POINT('',(99.6,14.9075133155355,90.032549368716));
#14082=CARTESIAN_POINT('',(0.4,26.4380602337443,94.8086582838175));
#14083=CARTESIAN_POINT('',(0.,26.4380602337443,94.8086582838175));
#14084=CARTESIAN_POINT('',(0.4,14.9075133155355,90.032549368716));
#14085=CARTESIAN_POINT('Origin',(99.8,14.9840500020085,89.8477734622137));
#14086=CARTESIAN_POINT('',(100.,26.3437390864656,94.3366323052791));
#14087=CARTESIAN_POINT('',(100.105946489469,26.4037529519037,94.2468152084245));
#14088=CARTESIAN_POINT('',(100.,26.9795649469519,94.6));
#14089=CARTESIAN_POINT('',(100.,15.0605866884815,89.6629975557115));
#14090=CARTESIAN_POINT('',(99.6956708580913,26.9190301168722,94.9043291419087));
#14091=CARTESIAN_POINT('',(100.,26.9795649469519,94.6));
#14092=CARTESIAN_POINT('',(96.6772607457411,11.7444577556222,91.8859190295585));
#14093=CARTESIAN_POINT('Origin',(99.75,12.7955266952966,81.1419733047034));
#14094=CARTESIAN_POINT('',(99.5,3.50355339059328,72.2035533905933));
#14095=CARTESIAN_POINT('',(99.5,12.61875,81.31875));
#14096=CARTESIAN_POINT('',(100.,3.65,71.6428932188134));
#14097=CARTESIAN_POINT('',(99.5,3.50355339059328,72.2035533905933));
#14098=CARTESIAN_POINT('',(100.,12.9723033905933,80.9651966094067));
#14099=CARTESIAN_POINT('Origin',(0.,26.9190301168722,94.9043291419087));
#14100=CARTESIAN_POINT('',(0.304329141908727,26.9190301168722,94.9043291419087));
#14101=CARTESIAN_POINT('',(1.48950104191211,20.9607686190275,93.7191572419054));
#14102=CARTESIAN_POINT('',(99.6,27.4,95.));
#14103=CARTESIAN_POINT('',(97.8609183745487,36.1429537356614,96.7390816254513));
#14104=CARTESIAN_POINT('',(0.4,27.4,95.));
#14105=CARTESIAN_POINT('',(0.,27.4,95.));
#14106=CARTESIAN_POINT('',(0.305843413104347,26.9266428722557,94.9058434131043));
#14107=CARTESIAN_POINT('Origin',(0.2,14.9840500020085,89.8477734622137));
#14108=CARTESIAN_POINT('',(0.,26.9795649469519,94.6));
#14109=CARTESIAN_POINT('',(-0.105946489468213,26.4037529519034,94.246815208425));
#14110=CARTESIAN_POINT('Origin',(0.2,27.0375,94.8));
#14111=CARTESIAN_POINT('',(0.4,34.4,95.));
#14112=CARTESIAN_POINT('',(0.4,27.0375,95.));
#14113=CARTESIAN_POINT('',(0.,34.2343145750508,94.6));
#14114=CARTESIAN_POINT('Origin',(99.75,25.,26.5));
#14115=CARTESIAN_POINT('',(100.,25.,28.55));
#14116=CARTESIAN_POINT('Origin',(100.,25.,26.5));
#14117=CARTESIAN_POINT('',(99.5,25.,28.05));
#14118=CARTESIAN_POINT('',(99.75,25.,28.3));
#14119=CARTESIAN_POINT('Origin',(99.5,25.,26.5));
#14120=CARTESIAN_POINT('Origin',(100.,19.075,47.5));
#14121=CARTESIAN_POINT('',(100.,3.65,61.0158240592278));
#14122=CARTESIAN_POINT('',(100.,3.65,59.675));
#14123=CARTESIAN_POINT('',(100.,3.65,33.9841759407722));
#14124=CARTESIAN_POINT('Origin',(100.,0.,47.5));
#14125=CARTESIAN_POINT('',(100.,3.65,14.4571067811865));
#14126=CARTESIAN_POINT('',(100.,3.65,59.675));
#14127=CARTESIAN_POINT('',(100.,13.3558711208215,4.751235660365));
#14128=CARTESIAN_POINT('',(100.,-0.827696609406725,18.9348033905933));
#14129=CARTESIAN_POINT('',(100.,13.4795649469519,4.7));
#14130=CARTESIAN_POINT('',(100.,8.21024487335069,6.88262383897043));
#14131=CARTESIAN_POINT('',(100.,22.1343145750508,4.7));
#14132=CARTESIAN_POINT('',(100.,16.0875,4.7));
#14133=CARTESIAN_POINT('',(100.,22.2,4.76568542494924));
#14134=CARTESIAN_POINT('',(100.,32.0859072875254,14.6515927124747));
#14135=CARTESIAN_POINT('',(100.,22.2,9.9));
#14136=CARTESIAN_POINT('',(100.,22.2,25.9));
#14137=CARTESIAN_POINT('',(100.,28.8,9.9));
#14138=CARTESIAN_POINT('',(100.,20.8375,9.9));
#14139=CARTESIAN_POINT('',(100.,28.8,0.765685424949241));
#14140=CARTESIAN_POINT('',(100.,28.8,28.5));
#14141=CARTESIAN_POINT('',(100.,29.1656854249492,0.4));
#14142=CARTESIAN_POINT('',(100.,14.7765927124746,14.7890927124745));
#14143=CARTESIAN_POINT('',(100.,34.2343145750507,0.4));
#14144=CARTESIAN_POINT('',(100.,23.7375,0.4));
#14145=CARTESIAN_POINT('',(100.,34.6,0.765685424949272));
#14146=CARTESIAN_POINT('',(100.,42.3109072875254,8.47659271247462));
#14147=CARTESIAN_POINT('',(100.,34.6,21.7343145750508));
#14148=CARTESIAN_POINT('',(100.,34.6,23.75));
#14149=CARTESIAN_POINT('',(100.,34.5343145750508,21.8));
#14150=CARTESIAN_POINT('',(100.,24.2609072875253,32.0734072875253));
#14151=CARTESIAN_POINT('',(100.,34.1,21.8));
#14152=CARTESIAN_POINT('',(100.,26.7875,21.8));
#14153=CARTESIAN_POINT('',(100.,34.1,73.3));
#14154=CARTESIAN_POINT('',(100.,34.1,60.2));
#14155=CARTESIAN_POINT('',(100.,34.5343145750508,73.3));
#14156=CARTESIAN_POINT('',(100.,27.5375,73.3));
#14157=CARTESIAN_POINT('',(100.,34.6,73.3656854249493));
#14158=CARTESIAN_POINT('',(100.,24.2359072875254,63.0015927124745));
#14159=CARTESIAN_POINT('',(100.,34.6,94.2343145750508));
#14160=CARTESIAN_POINT('',(100.,34.6,23.75));
#14161=CARTESIAN_POINT('',(100.,34.2343145750508,94.6));
#14162=CARTESIAN_POINT('',(100.,42.3109072875254,86.5234072875254));
#14163=CARTESIAN_POINT('',(100.,27.0375,94.6));
#14164=CARTESIAN_POINT('',(100.,25.,68.55));
#14165=CARTESIAN_POINT('Origin',(100.,25.,66.5));
#14166=CARTESIAN_POINT('Origin',(100.,25.,26.5));
#14167=CARTESIAN_POINT('',(92.,25.,28.05));
#14168=CARTESIAN_POINT('',(100.,25.,28.05));
#14169=CARTESIAN_POINT('Origin',(92.,25.,26.5));
#14170=CARTESIAN_POINT('Origin',(99.75,25.,66.5));
#14171=CARTESIAN_POINT('',(99.5,25.,68.05));
#14172=CARTESIAN_POINT('',(99.75,25.,68.3));
#14173=CARTESIAN_POINT('Origin',(99.5,25.,66.5));
#14174=CARTESIAN_POINT('Origin',(100.,25.,66.5));
#14175=CARTESIAN_POINT('',(92.,25.,68.05));
#14176=CARTESIAN_POINT('',(100.,25.,68.05));
#14177=CARTESIAN_POINT('Origin',(92.,25.,66.5));
#14178=CARTESIAN_POINT('Origin',(0.,3.65,71.6428932188134));
#14179=CARTESIAN_POINT('',(0.5,3.50355339059328,72.2035533905933));
#14180=CARTESIAN_POINT('',(0.5,3.15,71.35));
#14181=CARTESIAN_POINT('',(0.5,3.50355339059328,72.2035533905933));
#14182=CARTESIAN_POINT('',(0.,3.65,71.6428932188134));
#14183=CARTESIAN_POINT('',(0.5,3.15,71.35));
#14184=CARTESIAN_POINT('Origin',(0.25,12.7955266952966,81.1419733047034));
#14185=CARTESIAN_POINT('',(0.5,12.61875,81.31875));
#14186=CARTESIAN_POINT('Origin',(0.25,3.4,59.675));
#14187=CARTESIAN_POINT('',(0.5,3.15,61.1410226889336));
#14188=CARTESIAN_POINT('Origin',(3.65,0.,47.5));
#14189=CARTESIAN_POINT('',(0.5,3.15,59.675));
#14190=CARTESIAN_POINT('Origin',(99.5,3.15,71.35));
#14191=CARTESIAN_POINT('',(99.5,3.15,71.35));
#14192=CARTESIAN_POINT('',(99.5,3.15,71.35));
#14193=CARTESIAN_POINT('',(100.,3.65,71.6428932188134));
#14194=CARTESIAN_POINT('Origin',(0.,3.32677669529664,71.7767766952966));
#14195=CARTESIAN_POINT('',(0.,3.50355339059328,72.2035533905933));
#14196=CARTESIAN_POINT('',(0.,3.15,71.35));
#14197=CARTESIAN_POINT('Origin',(99.75,3.4,59.675));
#14198=CARTESIAN_POINT('',(99.5,3.15,61.1410226889336));
#14199=CARTESIAN_POINT('Origin',(96.3499999999999,0.,47.5));
#14200=CARTESIAN_POINT('',(99.5,3.15,59.675));
#14201=CARTESIAN_POINT('Origin',(0.,26.3,95.));
#14202=CARTESIAN_POINT('Origin',(0.5,3.50355339059327,13.8964466094067));
#14203=CARTESIAN_POINT('',(0.5,3.15,14.75));
#14204=CARTESIAN_POINT('',(0.,3.65,14.4571067811866));
#14205=CARTESIAN_POINT('',(0.5,3.50355339059327,13.8964466094067));
#14206=CARTESIAN_POINT('',(0.5,3.50355339059327,13.8964466094067));
#14207=CARTESIAN_POINT('',(0.5,3.15,14.75));
#14208=CARTESIAN_POINT('Origin',(0.25,-1.00447330470336,18.7580266952966));
#14209=CARTESIAN_POINT('',(0.4,13.1292893218813,4.41213203435597));
#14210=CARTESIAN_POINT('',(0.5,12.887867965644,4.51213203435597));
#14211=CARTESIAN_POINT('',(3.45785529853279,5.746973588389,7.4699873328888));
#14212=CARTESIAN_POINT('',(0.5,-1.18125,18.58125));
#14213=CARTESIAN_POINT('',(-0.48589817198775,13.6311103255984,5.16316024034552));
#14214=CARTESIAN_POINT('Origin',(99.5,3.50355339059327,13.8964466094067));
#14215=CARTESIAN_POINT('',(99.5,3.15,14.75));
#14216=CARTESIAN_POINT('',(99.5,3.15,14.75));
#14217=CARTESIAN_POINT('',(99.5,3.50355339059327,13.8964466094067));
#14218=CARTESIAN_POINT('',(99.5,3.50355339059327,13.8964466094067));
#14219=CARTESIAN_POINT('',(100.,3.65,14.4571067811865));
#14220=CARTESIAN_POINT('Origin',(0.,3.32677669529664,14.3232233047034));
#14221=CARTESIAN_POINT('',(0.,3.15,14.75));
#14222=CARTESIAN_POINT('',(0.,3.50355339059327,13.8964466094067));
#14223=CARTESIAN_POINT('Origin',(99.75,-1.00447330470336,18.7580266952966));
#14224=CARTESIAN_POINT('',(99.6,13.1292893218814,4.41213203435595));
#14225=CARTESIAN_POINT('',(100.485898171988,13.6311103255987,5.16316024034602));
#14226=CARTESIAN_POINT('',(99.5,12.887867965644,4.51213203435597));
#14227=CARTESIAN_POINT('',(99.5,-1.18125,18.58125));
#14228=CARTESIAN_POINT('',(90.1551656566029,-9.67255784431481,13.856966377753));
#14229=CARTESIAN_POINT('Origin',(99.75,3.4,59.675));
#14230=CARTESIAN_POINT('',(99.5,3.15,33.8589773110664));
#14231=CARTESIAN_POINT('Origin',(96.3499999999999,0.,47.5));
#14232=CARTESIAN_POINT('',(99.5,3.15,59.675));
#14233=CARTESIAN_POINT('Origin',(0.25,3.4,59.675));
#14234=CARTESIAN_POINT('',(0.5,3.15,33.8589773110664));
#14235=CARTESIAN_POINT('Origin',(3.65,0.,47.5));
#14236=CARTESIAN_POINT('',(0.5,3.15,59.675));
#14237=CARTESIAN_POINT('Origin',(0.,3.15,71.85));
#14238=CARTESIAN_POINT('',(0.,3.15,33.8589773110664));
#14239=CARTESIAN_POINT('',(77.5,3.15,19.));
#14240=CARTESIAN_POINT('Origin',(80.,3.15,19.));
#14241=CARTESIAN_POINT('',(47.5,3.15,19.));
#14242=CARTESIAN_POINT('Origin',(50.,3.15,19.));
#14243=CARTESIAN_POINT('',(17.5,3.15,19.));
#14244=CARTESIAN_POINT('Origin',(20.,3.15,19.));
#14245=CARTESIAN_POINT('Origin',(0.,0.,47.5));
#14246=CARTESIAN_POINT('',(0.,3.15,61.1410226889336));
#14247=CARTESIAN_POINT('Origin',(99.8,8.13370818687767,6.69784793246817));
#14248=CARTESIAN_POINT('',(99.6,13.4,4.3));
#14249=CARTESIAN_POINT('',(99.6,8.05717150040465,6.51307202596591));
#14250=CARTESIAN_POINT('',(100.,13.4795649469519,4.7));
#14251=CARTESIAN_POINT('Origin',(99.8,26.7875,22.));
#14252=CARTESIAN_POINT('',(99.6,34.7,22.2));
#14253=CARTESIAN_POINT('',(99.6,34.5,22.2));
#14254=CARTESIAN_POINT('',(99.6,26.7875,22.2));
#14255=CARTESIAN_POINT('',(99.6,34.5,22.2));
#14256=CARTESIAN_POINT('',(100.,34.5343145750508,21.8));
#14257=CARTESIAN_POINT('Origin',(99.8,27.0375,94.8));
#14258=CARTESIAN_POINT('',(99.6,34.4,95.));
#14259=CARTESIAN_POINT('',(100.,34.2343145750508,94.6));
#14260=CARTESIAN_POINT('',(99.6,27.0375,95.));
#14261=CARTESIAN_POINT('Origin',(99.8,42.4523286437627,86.6648286437627));
#14262=CARTESIAN_POINT('',(99.6,35.,94.4));
#14263=CARTESIAN_POINT('',(100.,34.6,94.2343145750508));
#14264=CARTESIAN_POINT('',(99.6,42.59375,86.80625));
#14265=CARTESIAN_POINT('Origin',(99.8,34.8,23.75));
#14266=CARTESIAN_POINT('',(99.6,35.,73.2));
#14267=CARTESIAN_POINT('',(100.,34.6,73.3656854249493));
#14268=CARTESIAN_POINT('',(99.6,35.,23.75));
#14269=CARTESIAN_POINT('Origin',(99.8,24.3773286437628,62.8601713562372));
#14270=CARTESIAN_POINT('',(99.6,34.7,72.9));
#14271=CARTESIAN_POINT('',(99.6,24.5187500000001,62.7187499999999));
#14272=CARTESIAN_POINT('',(100.,34.5343145750508,73.3));
#14273=CARTESIAN_POINT('Origin',(99.8,27.5375,73.1));
#14274=CARTESIAN_POINT('',(99.6,34.5,72.9));
#14275=CARTESIAN_POINT('',(99.6,27.5375,72.9));
#14276=CARTESIAN_POINT('',(100.,34.1,73.3));
#14277=CARTESIAN_POINT('Origin',(99.8,34.3,60.2));
#14278=CARTESIAN_POINT('',(99.6,34.5,60.2));
#14279=CARTESIAN_POINT('Origin',(99.8,24.4023286437626,32.2148286437626));
#14280=CARTESIAN_POINT('',(99.6,35.,21.9));
#14281=CARTESIAN_POINT('',(99.6,24.5437499999999,32.3562499999999));
#14282=CARTESIAN_POINT('',(100.,34.6,21.7343145750508));
#14283=CARTESIAN_POINT('Origin',(99.8,34.8,23.75));
#14284=CARTESIAN_POINT('',(99.6,35.,0.6));
#14285=CARTESIAN_POINT('',(99.6,35.,23.75));
#14286=CARTESIAN_POINT('',(100.,34.6,0.765685424949275));
#14287=CARTESIAN_POINT('Origin',(99.8,42.4523286437627,8.33517135623731));
#14288=CARTESIAN_POINT('',(99.6,34.4,0.));
#14289=CARTESIAN_POINT('',(99.6,42.59375,8.19374999999999));
#14290=CARTESIAN_POINT('',(100.,34.2343145750507,0.4));
#14291=CARTESIAN_POINT('Origin',(99.8,23.7375,0.2));
#14292=CARTESIAN_POINT('',(99.6,29.,0.));
#14293=CARTESIAN_POINT('',(99.6,23.7375,0.));
#14294=CARTESIAN_POINT('',(100.,29.1656854249492,0.4));
#14295=CARTESIAN_POINT('Origin',(99.8,14.6351713562373,14.6476713562372));
#14296=CARTESIAN_POINT('',(99.6,28.4,0.6));
#14297=CARTESIAN_POINT('',(99.6,14.49375,14.5062499999999));
#14298=CARTESIAN_POINT('',(100.,28.8,0.765685424949241));
#14299=CARTESIAN_POINT('Origin',(99.8,28.6,28.5));
#14300=CARTESIAN_POINT('',(99.6,28.4,9.5));
#14301=CARTESIAN_POINT('',(99.6,28.4,28.5));
#14302=CARTESIAN_POINT('',(100.,28.8,9.9));
#14303=CARTESIAN_POINT('Origin',(99.8,20.8375,9.7));
#14304=CARTESIAN_POINT('',(99.6,22.6,9.5));
#14305=CARTESIAN_POINT('',(99.6,20.8375,9.5));
#14306=CARTESIAN_POINT('',(100.,22.2,9.9));
#14307=CARTESIAN_POINT('Origin',(99.8,22.4,25.9));
#14308=CARTESIAN_POINT('',(99.6,22.6,4.6));
#14309=CARTESIAN_POINT('',(99.6,22.6,25.9));
#14310=CARTESIAN_POINT('',(100.,22.2,4.76568542494924));
#14311=CARTESIAN_POINT('Origin',(99.8,32.2273286437627,14.5101713562374));
#14312=CARTESIAN_POINT('',(99.6,22.3,4.3));
#14313=CARTESIAN_POINT('',(99.6,32.36875,14.3687500000001));
#14314=CARTESIAN_POINT('',(100.,22.1343145750508,4.7));
#14315=CARTESIAN_POINT('Origin',(99.8,16.0875,4.5));
#14316=CARTESIAN_POINT('',(99.6,16.0875,4.3));
#14317=CARTESIAN_POINT('Origin',(0.,28.7,0.3));
#14318=CARTESIAN_POINT('',(0.4,28.4,0.6));
#14319=CARTESIAN_POINT('',(0.,28.4,0.6));
#14320=CARTESIAN_POINT('',(0.4,29.,0.));
#14321=CARTESIAN_POINT('',(0.4,14.49375,14.5062499999999));
#14322=CARTESIAN_POINT('',(0.,29.,0.));
#14323=CARTESIAN_POINT('Origin',(0.,28.4,9.5));
#14324=CARTESIAN_POINT('',(0.4,28.4,9.5));
#14325=CARTESIAN_POINT('',(0.,28.4,9.5));
#14326=CARTESIAN_POINT('',(0.4,28.4,28.5));
#14327=CARTESIAN_POINT('Origin',(0.,22.6,9.5));
#14328=CARTESIAN_POINT('',(0.4,22.6,9.5));
#14329=CARTESIAN_POINT('',(0.,22.6,9.5));
#14330=CARTESIAN_POINT('',(0.4,20.8375,9.5));
#14331=CARTESIAN_POINT('Origin',(0.,22.6,4.3));
#14332=CARTESIAN_POINT('',(0.4,22.6,4.6));
#14333=CARTESIAN_POINT('',(0.,22.6,4.6));
#14334=CARTESIAN_POINT('',(0.4,22.6,25.9));
#14335=CARTESIAN_POINT('Origin',(0.,22.45,4.45));
#14336=CARTESIAN_POINT('',(0.4,22.3,4.3));
#14337=CARTESIAN_POINT('',(0.,22.3,4.3));
#14338=CARTESIAN_POINT('',(0.4,32.36875,14.3687500000001));
#14339=CARTESIAN_POINT('Origin',(0.,13.1,4.3));
#14340=CARTESIAN_POINT('',(0.4,13.4,4.3));
#14341=CARTESIAN_POINT('',(0.,13.4,4.3));
#14342=CARTESIAN_POINT('',(0.4,16.0875,4.3));
#14343=CARTESIAN_POINT('Origin',(0.,13.143933982822,4.40606601717798));
#14344=CARTESIAN_POINT('',(0.4,8.05717150040465,6.51307202596591));
#14345=CARTESIAN_POINT('',(0.,12.887867965644,4.51213203435597));
#14346=CARTESIAN_POINT('Origin',(0.,3.15,14.25));
#14347=CARTESIAN_POINT('Origin',(0.2,8.13370818687767,6.69784793246817));
#14348=CARTESIAN_POINT('',(0.,13.4795649469519,4.7));
#14349=CARTESIAN_POINT('Origin',(0.2,16.0875,4.5));
#14350=CARTESIAN_POINT('',(0.,22.1343145750508,4.7));
#14351=CARTESIAN_POINT('Origin',(0.2,32.2273286437627,14.5101713562374));
#14352=CARTESIAN_POINT('',(0.,22.2,4.76568542494924));
#14353=CARTESIAN_POINT('Origin',(0.2,22.4,25.9));
#14354=CARTESIAN_POINT('',(0.,22.2,9.9));
#14355=CARTESIAN_POINT('Origin',(0.2,20.8375,9.7));
#14356=CARTESIAN_POINT('',(0.,28.8,9.9));
#14357=CARTESIAN_POINT('Origin',(0.2,28.6,28.5));
#14358=CARTESIAN_POINT('',(0.,28.8,0.765685424949238));
#14359=CARTESIAN_POINT('Origin',(0.2,14.6351713562373,14.6476713562372));
#14360=CARTESIAN_POINT('',(0.,29.1656854249492,0.4));
#14361=CARTESIAN_POINT('Origin',(0.2,23.7375,0.2));
#14362=CARTESIAN_POINT('',(0.4,34.4,0.));
#14363=CARTESIAN_POINT('',(0.,34.2343145750507,0.400000000000001));
#14364=CARTESIAN_POINT('',(0.4,23.7375,0.));
#14365=CARTESIAN_POINT('Origin',(0.2,42.4523286437627,8.33517135623731));
#14366=CARTESIAN_POINT('',(0.4,35.,0.6));
#14367=CARTESIAN_POINT('',(0.,34.6,0.765685424949272));
#14368=CARTESIAN_POINT('',(0.4,42.59375,8.19374999999999));
#14369=CARTESIAN_POINT('Origin',(0.2,34.8,23.75));
#14370=CARTESIAN_POINT('',(0.4,35.,21.9));
#14371=CARTESIAN_POINT('',(0.,34.6,21.7343145750508));
#14372=CARTESIAN_POINT('',(0.4,35.,23.75));
#14373=CARTESIAN_POINT('Origin',(0.2,24.4023286437626,32.2148286437626));
#14374=CARTESIAN_POINT('',(0.4,34.7,22.2));
#14375=CARTESIAN_POINT('',(0.,34.5343145750508,21.8));
#14376=CARTESIAN_POINT('',(0.4,24.5437499999999,32.3562499999999));
#14377=CARTESIAN_POINT('Origin',(0.2,26.7875,22.));
#14378=CARTESIAN_POINT('',(0.4,34.5,22.2));
#14379=CARTESIAN_POINT('',(0.,34.1,21.8));
#14380=CARTESIAN_POINT('',(0.4,26.7875,22.2));
#14381=CARTESIAN_POINT('Origin',(0.2,27.5375,73.1));
#14382=CARTESIAN_POINT('',(0.4,34.7,72.9));
#14383=CARTESIAN_POINT('',(0.,34.5343145750508,73.3));
#14384=CARTESIAN_POINT('',(0.4,34.5,72.9));
#14385=CARTESIAN_POINT('',(0.4,27.5375,72.9));
#14386=CARTESIAN_POINT('',(0.4,34.5,72.9));
#14387=CARTESIAN_POINT('Origin',(0.2,24.3773286437628,62.8601713562372));
#14388=CARTESIAN_POINT('',(0.4,35.,73.2));
#14389=CARTESIAN_POINT('',(0.4,24.5187500000001,62.7187499999999));
#14390=CARTESIAN_POINT('',(0.,34.6,73.3656854249492));
#14391=CARTESIAN_POINT('Origin',(0.2,34.8,23.75));
#14392=CARTESIAN_POINT('',(0.4,35.,94.4));
#14393=CARTESIAN_POINT('',(0.4,35.,23.75));
#14394=CARTESIAN_POINT('',(0.,34.6,94.2343145750508));
#14395=CARTESIAN_POINT('Origin',(0.2,34.3,60.2));
#14396=CARTESIAN_POINT('',(0.4,34.5,60.2));
#14397=CARTESIAN_POINT('Origin',(0.2,42.4523286437627,86.6648286437627));
#14398=CARTESIAN_POINT('',(0.4,42.59375,86.80625));
#14399=CARTESIAN_POINT('Origin',(0.,28.4,0.));
#14400=CARTESIAN_POINT('',(0.,34.4,0.));
#14401=CARTESIAN_POINT('Origin',(0.,34.7,0.3));
#14402=CARTESIAN_POINT('',(0.,35.,0.6));
#14403=CARTESIAN_POINT('Origin',(0.,35.,0.));
#14404=CARTESIAN_POINT('',(0.,35.,21.9));
#14405=CARTESIAN_POINT('',(17.5,35.,19.));
#14406=CARTESIAN_POINT('Origin',(20.,35.,19.));
#14407=CARTESIAN_POINT('',(47.5,35.,19.));
#14408=CARTESIAN_POINT('Origin',(50.,35.,19.));
#14409=CARTESIAN_POINT('',(77.5,35.,19.));
#14410=CARTESIAN_POINT('Origin',(80.,35.,19.));
#14411=CARTESIAN_POINT('Origin',(0.,34.85,22.05));
#14412=CARTESIAN_POINT('',(0.,34.7,22.2));
#14413=CARTESIAN_POINT('Origin',(0.,34.5,22.2));
#14414=CARTESIAN_POINT('',(0.,34.5,22.2));
#14415=CARTESIAN_POINT('Origin',(0.,34.5,72.9));
#14416=CARTESIAN_POINT('',(0.,34.5,72.9));
#14417=CARTESIAN_POINT('Origin',(0.,36.,72.9));
#14418=CARTESIAN_POINT('',(0.,34.7,72.9));
#14419=CARTESIAN_POINT('Origin',(0.,34.85,73.05));
#14420=CARTESIAN_POINT('',(0.,35.,73.2));
#14421=CARTESIAN_POINT('Origin',(0.,35.,0.));
#14422=CARTESIAN_POINT('',(0.,35.,94.4));
#14423=CARTESIAN_POINT('Origin',(0.,34.7,94.7));
#14424=CARTESIAN_POINT('',(0.,34.4,95.));
#14425=CARTESIAN_POINT('Origin',(0.,35.,95.));
#14426=CARTESIAN_POINT('Origin',(92.,25.,26.5));
#14427=CARTESIAN_POINT('Origin',(92.,25.,66.5));
#14428=CARTESIAN_POINT('Origin',(8.,25.,26.5));
#14429=CARTESIAN_POINT('Origin',(8.,25.,66.5));
#14430=CARTESIAN_POINT('Origin',(20.,35.,19.));
#14431=CARTESIAN_POINT('',(17.5,35.,19.));
#14432=CARTESIAN_POINT('Origin',(50.,35.,19.));
#14433=CARTESIAN_POINT('',(47.5,35.,19.));
#14434=CARTESIAN_POINT('Origin',(80.,35.,19.));
#14435=CARTESIAN_POINT('',(77.5,35.,19.));
#14436=CARTESIAN_POINT('Origin',(0.,3.15,71.85));
#18257=UNCERTAINTY_MEASURE_WITH_UNIT(LENGTH_MEASURE(0.01),#18282,
'DISTANCE_ACCURACY_VALUE',
'Maximum model space distance between geometric entities at asserted c
onnectivities');
#18266=UNCERTAINTY_MEASURE_WITH_UNIT(LENGTH_MEASURE(0.01),#18282,
'DISTANCE_ACCURACY_VALUE',
'Maximum model space distance between geometric entities at asserted c
onnectivities');
#18272=(
GEOMETRIC_REPRESENTATION_CONTEXT(3)
GLOBAL_UNCERTAINTY_ASSIGNED_CONTEXT((#18257))
GLOBAL_UNIT_ASSIGNED_CONTEXT((#18282,#18284,#18285))
REPRESENTATION_CONTEXT('','3D')
);
#18281=(
GEOMETRIC_REPRESENTATION_CONTEXT(3)
GLOBAL_UNCERTAINTY_ASSIGNED_CONTEXT((#18266))
GLOBAL_UNIT_ASSIGNED_CONTEXT((#18282,#18284,#18285))
REPRESENTATION_CONTEXT('','3D')
);
#18282=(
LENGTH_UNIT()
NAMED_UNIT(*)
SI_UNIT(.MILLI.,.METRE.)
);
#18284=(
NAMED_UNIT(*)
PLANE_ANGLE_UNIT()
SI_UNIT($,.RADIAN.)
);
#18285=(
NAMED_UNIT(*)
SI_UNIT($,.STERADIAN.)
SOLID_ANGLE_UNIT()
);
#18291=SHAPE_DEFINITION_REPRESENTATION(#18305,#18343);
#18305=PRODUCT_DEFINITION_SHAPE('',$,#18358);
#18343=SHAPE_REPRESENTATION('',(#9544),#18272);
#18352=PRODUCT_DEFINITION_CONTEXT('part definition',#18396,'design');
#18358=PRODUCT_DEFINITION('2026-10-20-13-03-16-349',
'01_Pole_Block_Steel',#18372,#18352);
#18372=PRODUCT_DEFINITION_FORMATION('',$,#18403);
#18396=APPLICATION_CONTEXT(
'Core Data for Automotive Mechanical Design Process');
#18397=PRODUCT_CONTEXT('part definition',#18396,'mechanical');
#18403=PRODUCT('2026-10-20-13-03-16-349','01_Pole_Block_Steel',$,(#18397));
#18447=COLOUR_RGB('Dark Blue',0.08,0.2,0.34);
#18448=FILL_AREA_STYLE_COLOUR('',#18447);
#18449=FILL_AREA_STYLE('',(#18448));
#18450=SURFACE_STYLE_FILL_AREA(#18449);
#18451=SURFACE_SIDE_STYLE('',(#18450));
#18452=SURFACE_STYLE_USAGE(.BOTH.,#18451);
#18453=PRESENTATION_STYLE_ASSIGNMENT((#18452));
ENDSEC;
END-ISO-10303-21;
